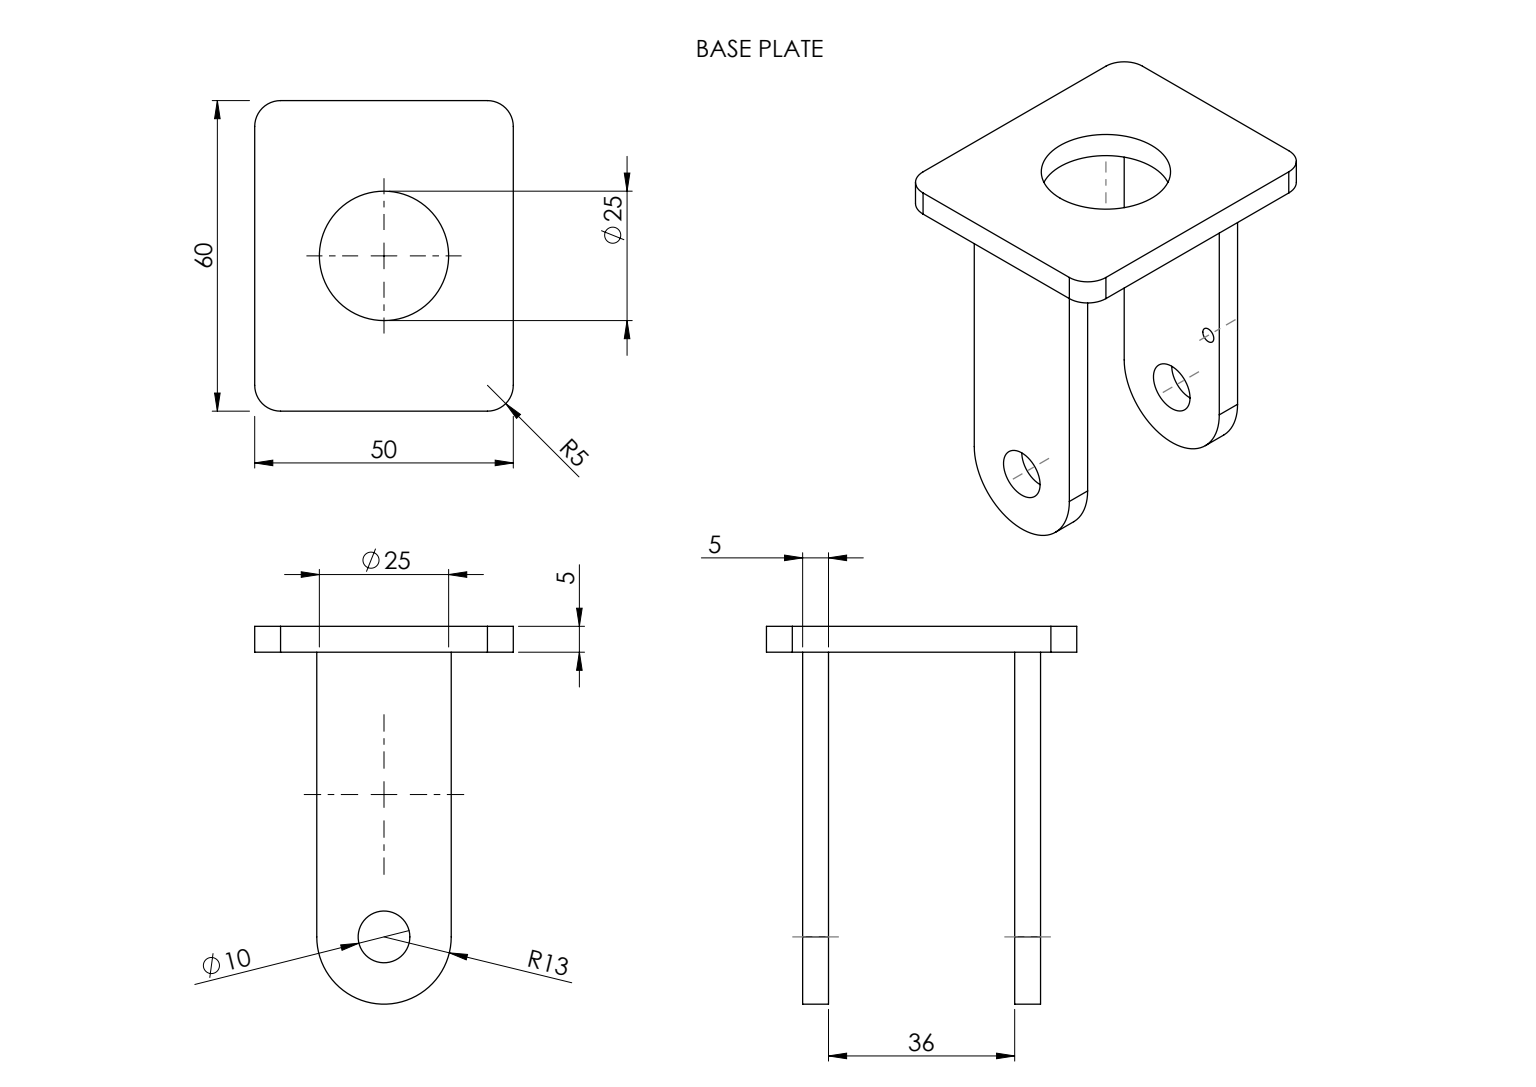
ISO-10303-21;
HEADER;
FILE_DESCRIPTION (('STEP AP214'),
    '1' );
FILE_NAME ('base plate.step',
    '2026-09-30T16:28:02',
    ( '' ),
    ( '' ),
    'SwSTEP 2.0',
    'SolidWorks 2026',
    '' );
FILE_SCHEMA (( 'AUTOMOTIVE_DESIGN' ));
ENDSEC;

DATA;
#4=PLANE ( 'NONE',  #18463 ) ;
#89=DIRECTION ( 'NONE',  ( -1.000000000000000000, 2.207829878515935943E-16, 0.000000000000000000 ) ) ;
#94=CARTESIAN_POINT ( 'NONE',  ( -13.00000000000001243, 55.00000000000000711, 18.00000000000000000 ) ) ;
#112=AXIS2_PLACEMENT_3D ( 'NONE', #25183, #25333, #20434 ) ;
#150=DIRECTION ( 'NONE',  ( 0.000000000000000000, -0.000000000000000000, -1.000000000000000000 ) ) ;
#243=( NAMED_UNIT ( * ) PLANE_ANGLE_UNIT ( ) SI_UNIT ( $, .RADIAN. ) );
#303=EDGE_CURVE ( 'NONE', #13765, #18617, #4330, .T. ) ;
#312=ORIENTED_EDGE ( 'NONE', *, *, #15522, .T. ) ;
#351=PLANE ( 'NONE',  #28566 ) ;
#361=DIRECTION ( 'NONE',  ( 0.000000000000000000, -1.000000000000000000, 0.000000000000000000 ) ) ;
#433=CARTESIAN_POINT ( 'NONE',  ( -13.00000000000001243, 55.00000000000000711, -23.00000000000000000 ) ) ;
#466=ORIENTED_EDGE ( 'NONE', *, *, #9296, .T. ) ;
#467=EDGE_CURVE ( 'NONE', #22249, #23534, #732, .T. ) ;
#553=DIRECTION ( 'NONE',  ( -0.000000000000000000, -1.000000000000000000, -0.000000000000000000 ) ) ;
#578=AXIS2_PLACEMENT_3D ( 'NONE', #20455, #15424, #27383 ) ;
#597=DIRECTION ( 'NONE',  ( -2.207829878515935943E-16, 1.000000000000000000, 0.000000000000000000 ) ) ;
#643=DIRECTION ( 'NONE',  ( 0.000000000000000000, -1.000000000000000000, 0.000000000000000000 ) ) ;
#651=ORIENTED_EDGE ( 'NONE', *, *, #17517, .T. ) ;
#653=VERTEX_POINT ( 'NONE', #12872 ) ;
#675=DIRECTION ( 'NONE',  ( -0.000000000000000000, 1.000000000000000000, -0.000000000000000000 ) ) ;
#732=LINE ( 'NONE', #12472, #2865 ) ;
#752=CARTESIAN_POINT ( 'NONE',  ( 19.99999999999998934, 55.00000000000000711, -30.00000000000000000 ) ) ;
#753=ORIENTED_EDGE ( 'NONE', *, *, #7733, .T. ) ;
#775=EDGE_CURVE ( 'NONE', #20254, #13743, #1148, .T. ) ;
#790=CARTESIAN_POINT ( 'NONE',  ( 0.000000000000000000, 0.000000000000000000, 23.00000000000000000 ) ) ;
#820=AXIS2_PLACEMENT_3D ( 'NONE', #9199, #2219, #20356 ) ;
#827=AXIS2_PLACEMENT_3D ( 'NONE', #15460, #13176, #18050 ) ;
#846=VERTEX_POINT ( 'NONE', #9130 ) ;
#852=ORIENTED_EDGE ( 'NONE', *, *, #16824, .T. ) ;
#873=DIRECTION ( 'NONE',  ( 0.000000000000000000, 0.000000000000000000, 1.000000000000000000 ) ) ;
#883=CARTESIAN_POINT ( 'NONE',  ( -24.99999999999999289, 60.00000000000000711, -30.00000000000000711 ) ) ;
#951=EDGE_CURVE ( 'NONE', #20254, #12966, #17007, .T. ) ;
#1021=( NAMED_UNIT ( * ) PLANE_ANGLE_UNIT ( ) SI_UNIT ( $, .RADIAN. ) );
#1050=ORIENTED_EDGE ( 'NONE', *, *, #15240, .T. ) ;
#1103=VECTOR ( 'NONE', #29704, 1000.000000000000000 ) ;
#1148=LINE ( 'NONE', #3294, #1929 ) ;
#1209=DIRECTION ( 'NONE',  ( -1.387778780781445922E-16, 0.000000000000000000, 1.000000000000000000 ) ) ;
#1239=EDGE_CURVE ( 'NONE', #12966, #20254, #11655, .T. ) ;
#1281=DIRECTION ( 'NONE',  ( -0.000000000000000000, -0.000000000000000000, 1.000000000000000000 ) ) ;
#1304=ADVANCED_FACE ( 'NONE', ( #10036 ), #15218, .F. ) ;
#1305=ORIENTED_EDGE ( 'NONE', *, *, #467, .F. ) ;
#1362=FACE_OUTER_BOUND ( 'NONE', #5538, .T. ) ;
#1413=CARTESIAN_POINT ( 'NONE',  ( 20.00000000000000711, 60.00000000000000711, 29.99999999999998579 ) ) ;
#1433=CARTESIAN_POINT ( 'NONE',  ( 0.000000000000000000, 0.000000000000000000, -23.00000000000000000 ) ) ;
#1502=EDGE_LOOP ( 'NONE', ( #15115, #4598, #15245, #10391 ) ) ;
#1512=AXIS2_PLACEMENT_3D ( 'NONE', #12480, #12790, #7761 ) ;
#1514=LINE ( 'NONE', #20110, #6493 ) ;
#1535=PLANE ( 'NONE',  #25718 ) ;
#1601=LINE ( 'NONE', #10877, #8584 ) ;
#1665=EDGE_CURVE ( 'NONE', #3391, #13743, #22398, .T. ) ;
#1666=CARTESIAN_POINT ( 'NONE',  ( -24.99999999999998934, 55.00000000000000711, 29.99999999999999289 ) ) ;
#1684=LINE ( 'NONE', #13564, #22276 ) ;
#1775=VECTOR ( 'NONE', #13954, 1000.000000000000000 ) ;
#1791=DIRECTION ( 'NONE',  ( -0.000000000000000000, 1.000000000000000000, -0.000000000000000000 ) ) ;
#1812=CARTESIAN_POINT ( 'NONE',  ( -24.99999999999998934, 55.00000000000000711, 24.99999999999998934 ) ) ;
#1837=EDGE_CURVE ( 'NONE', #23534, #6999, #8618, .T. ) ;
#1921=CARTESIAN_POINT ( 'NONE',  ( -19.99999999999998934, 60.00000000000000711, 29.99999999999999289 ) ) ;
#1928=LINE ( 'NONE', #13648, #29476 ) ;
#1929=VECTOR ( 'NONE', #5267, 1000.000000000000000 ) ;
#1988=CARTESIAN_POINT ( 'NONE',  ( 8.469702402841419307E-15, 55.00000000000000711, 12.49999999999999112 ) ) ;
#2054=DIRECTION ( 'NONE',  ( 0.000000000000000000, 0.000000000000000000, -1.000000000000000000 ) ) ;
#2059=ORIENTED_EDGE ( 'NONE', *, *, #8323, .T. ) ;
#2102=AXIS2_PLACEMENT_3D ( 'NONE', #21046, #150, #16913 ) ;
#2147=DIRECTION ( 'NONE',  ( 0.000000000000000000, 0.000000000000000000, -1.000000000000000000 ) ) ;
#2163=ORIENTED_EDGE ( 'NONE', *, *, #14056, .F. ) ;
#2218=EDGE_CURVE ( 'NONE', #19798, #4416, #26479, .T. ) ;
#2219=DIRECTION ( 'NONE',  ( 0.000000000000000000, -1.000000000000000000, 0.000000000000000000 ) ) ;
#2237=( LENGTH_UNIT ( ) NAMED_UNIT ( * ) SI_UNIT ( .MILLI., .METRE. ) );
#2268=AXIS2_PLACEMENT_3D ( 'NONE', #28367, #7860, #2691 ) ;
#2305=ADVANCED_FACE ( 'NONE', ( #10419 ), #19581, .F. ) ;
#2341=DIRECTION ( 'NONE',  ( -1.000000000000000000, 0.000000000000000000, 1.387778780781445676E-16 ) ) ;
#2364=CYLINDRICAL_SURFACE ( 'NONE', #20773, 13.00000000000000178 ) ;
#2387=ADVANCED_FACE ( 'NONE', ( #8725 ), #10727, .F. ) ;
#2401=CARTESIAN_POINT ( 'NONE',  ( 13.00000000000001243, 55.00000000000000711, 18.00000000000000000 ) ) ;
#2495=EDGE_CURVE ( 'NONE', #18617, #28674, #20327, .T. ) ;
#2518=CARTESIAN_POINT ( 'NONE',  ( -13.00000000000000178, -2.870178842070716726E-15, -18.00000000000000000 ) ) ;
#2527=CARTESIAN_POINT ( 'NONE',  ( 0.000000000000000000, 0.000000000000000000, -23.00000000000000000 ) ) ;
#2554=ORIENTED_EDGE ( 'NONE', *, *, #28546, .F. ) ;
#2586=CIRCLE ( 'NONE', #11332, 5.000000000000000888 ) ;
#2630=DIRECTION ( 'NONE',  ( -1.000000000000000000, -2.207829878515935943E-16, 0.000000000000000000 ) ) ;
#2640=FACE_BOUND ( 'NONE', #22846, .T. ) ;
#2691=DIRECTION ( 'NONE',  ( 6.938893903907226800E-15, 0.000000000000000000, -1.000000000000000000 ) ) ;
#2739=VECTOR ( 'NONE', #10171, 1000.000000000000000 ) ;
#2788=CIRCLE ( 'NONE', #23227, 5.000000000000000000 ) ;
#2793=DIRECTION ( 'NONE',  ( -0.000000000000000000, 0.000000000000000000, 1.000000000000000000 ) ) ;
#2865=VECTOR ( 'NONE', #597, 1000.000000000000000 ) ;
#2897=ADVANCED_FACE ( 'NONE', ( #26440 ), #17257, .T. ) ;
#2982=DIRECTION ( 'NONE',  ( 0.000000000000000000, 0.000000000000000000, -1.000000000000000000 ) ) ;
#2988=CARTESIAN_POINT ( 'NONE',  ( 13.00000000000000178, -2.870178842070716726E-15, 23.00000000000000000 ) ) ;
#3027=DIRECTION ( 'NONE',  ( 0.000000000000000000, -1.000000000000000000, -0.000000000000000000 ) ) ;
#3040=ADVANCED_FACE ( 'NONE', ( #7024, #21193 ), #4, .F. ) ;
#3047=DIRECTION ( 'NONE',  ( 1.000000000000000000, 0.000000000000000000, 0.000000000000000000 ) ) ;
#3050=DIRECTION ( 'NONE',  ( 0.000000000000000000, -1.000000000000000000, 0.000000000000000000 ) ) ;
#3065=CARTESIAN_POINT ( 'NONE',  ( 13.00000000000001243, 55.00000000000000711, -23.00000000000000000 ) ) ;
#3163=( LENGTH_UNIT ( ) NAMED_UNIT ( * ) SI_UNIT ( .MILLI., .METRE. ) );
#3232=PRODUCT_CONTEXT ( 'NONE', #11423, 'mechanical' ) ;
#3236=COLOUR_RGB ( '', 0.09019608, 0.27058824, 0.51372549) ;
#3274=AXIS2_PLACEMENT_3D ( 'NONE', #13005, #17580, #15441 ) ;
#3285=CARTESIAN_POINT ( 'NONE',  ( -5.000000000000000000, 0.000000000000000000, -23.00000000000000000 ) ) ;
#3291=ORIENTED_EDGE ( 'NONE', *, *, #21767, .F. ) ;
#3294=CARTESIAN_POINT ( 'NONE',  ( 8.469702402841419307E-15, 60.00000000000000711, 12.49999999999999112 ) ) ;
#3295=LINE ( 'NONE', #19892, #25365 ) ;
#3296=CIRCLE ( 'NONE', #20319, 1.499999999999996225 ) ;
#3349=LINE ( 'NONE', #10189, #11351 ) ;
#3350=CARTESIAN_POINT ( 'NONE',  ( 6.938893903907228378E-15, 60.00000000000000711, -1.040834085586084257E-14 ) ) ;
#3369=ORIENTED_EDGE ( 'NONE', *, *, #4832, .F. ) ;
#3391=VERTEX_POINT ( 'NONE', #24824 ) ;
#3430=DIRECTION ( 'NONE',  ( 1.000000000000000000, 0.000000000000000000, 0.000000000000000000 ) ) ;
#3463=DIRECTION ( 'NONE',  ( 1.000000000000000000, 0.000000000000000000, 0.000000000000000000 ) ) ;
#3477=ADVANCED_FACE ( 'NONE', ( #25560 ), #5110, .F. ) ;
#3497=DIRECTION ( 'NONE',  ( 1.000000000000000000, 0.000000000000000000, 1.387778780781445922E-16 ) ) ;
#3515=CARTESIAN_POINT ( 'NONE',  ( 13.00000000000000178, -2.870178842070716726E-15, 23.00000000000000000 ) ) ;
#3527=VECTOR ( 'NONE', #675, 1000.000000000000000 ) ;
#3535=ORIENTED_EDGE ( 'NONE', *, *, #29533, .T. ) ;
#3543=AXIS2_PLACEMENT_3D ( 'NONE', #15895, #13310, #22633 ) ;
#3550=EDGE_LOOP ( 'NONE', ( #25606, #8516, #3369, #29957 ) ) ;
#3565=ORIENTED_EDGE ( 'NONE', *, *, #25043, .T. ) ;
#3584=LINE ( 'NONE', #22188, #8766 ) ;
#3613=CARTESIAN_POINT ( 'NONE',  ( 10.00000000000008527, 17.32050807568872486, -30.00000000000000711 ) ) ;
#3645=EDGE_CURVE ( 'NONE', #27580, #29940, #3295, .T. ) ;
#3670=CARTESIAN_POINT ( 'NONE',  ( -13.00000000000001243, 55.00000000000000711, 23.00000000000000000 ) ) ;
#3687=ORIENTED_EDGE ( 'NONE', *, *, #24489, .F. ) ;
#3776=CARTESIAN_POINT ( 'NONE',  ( -13.00000000000000178, -2.870178842070716726E-15, -18.00000000000000000 ) ) ;
#3785=ADVANCED_FACE ( 'NONE', ( #11184 ), #8445, .T. ) ;
#3815=DIRECTION ( 'NONE',  ( -0.000000000000000000, 1.000000000000000000, -0.000000000000000000 ) ) ;
#3841=CARTESIAN_POINT ( 'NONE',  ( 25.00000000000000000, 55.00000000000000711, -24.99999999999999289 ) ) ;
#3862=EDGE_CURVE ( 'NONE', #15686, #5157, #11281, .T. ) ;
#3942=( GEOMETRIC_REPRESENTATION_CONTEXT ( 3 ) GLOBAL_UNCERTAINTY_ASSIGNED_CONTEXT ( ( #30012 ) ) GLOBAL_UNIT_ASSIGNED_CONTEXT ( ( #3163, #10603, #21756 ) ) REPRESENTATION_CONTEXT ( 'NONE', 'WORKASPACE' ) );
#3978=DIRECTION ( 'NONE',  ( -0.000000000000000000, -0.000000000000000000, 1.000000000000000000 ) ) ;
#3985=VERTEX_POINT ( 'NONE', #10993 ) ;
#3989=EDGE_CURVE ( 'NONE', #13765, #14128, #27497, .T. ) ;
#4003=VECTOR ( 'NONE', #1281, 1000.000000000000000 ) ;
#4052=EDGE_LOOP ( 'NONE', ( #28141, #29867, #12630, #29986 ) ) ;
#4093=DIRECTION ( 'NONE',  ( 1.000000000000000000, 0.000000000000000000, -1.387778780781445676E-16 ) ) ;
#4112=DIRECTION ( 'NONE',  ( -0.000000000000000000, -0.000000000000000000, 1.000000000000000000 ) ) ;
#4160=EDGE_CURVE ( 'NONE', #13649, #22275, #16289, .T. ) ;
#4162=ORIENTED_EDGE ( 'NONE', *, *, #15722, .T. ) ;
#4184=ADVANCED_FACE ( 'NONE', ( #11711 ), #18889, .F. ) ;
#4330=CIRCLE ( 'NONE', #21386, 13.00000000000000178 ) ;
#4372=VECTOR ( 'NONE', #5031, 1000.000000000000000 ) ;
#4393=VECTOR ( 'NONE', #13496, 1000.000000000000000 ) ;
#4416=VERTEX_POINT ( 'NONE', #26691 ) ;
#4431=CARTESIAN_POINT ( 'NONE',  ( 0.000000000000000000, 0.000000000000000000, 18.00000000000000000 ) ) ;
#4432=CARTESIAN_POINT ( 'NONE',  ( 13.00000000000001243, 55.00000000000000711, -23.00000000000000000 ) ) ;
#4500=CARTESIAN_POINT ( 'NONE',  ( -24.99999999999998934, 55.00000000000000711, 29.99999999999999289 ) ) ;
#4511=SURFACE_STYLE_FILL_AREA ( #18392 ) ;
#4521=FACE_BOUND ( 'NONE', #26367, .T. ) ;
#4598=ORIENTED_EDGE ( 'NONE', *, *, #12300, .F. ) ;
#4649=CIRCLE ( 'NONE', #19739, 1.499999999999996225 ) ;
#4662=ADVANCED_FACE ( 'NONE', ( #7137, #23312 ), #23468, .F. ) ;
#4688=DIRECTION ( 'NONE',  ( 0.000000000000000000, 0.000000000000000000, -1.000000000000000000 ) ) ;
#4708=AXIS2_PLACEMENT_3D ( 'NONE', #17140, #9953, #14831 ) ;
#4743=CARTESIAN_POINT ( 'NONE',  ( -24.99999999999999289, 60.00000000000000711, -25.00000000000000000 ) ) ;
#4832=EDGE_CURVE ( 'NONE', #17767, #27247, #22973, .T. ) ;
#4914=CARTESIAN_POINT ( 'NONE',  ( -13.00000000000000178, -2.870178842070716726E-15, 23.00000000000000000 ) ) ;
#4918=AXIS2_PLACEMENT_3D ( 'NONE', #23936, #3027, #22224 ) ;
#5008=VERTEX_POINT ( 'NONE', #15798 ) ;
#5031=DIRECTION ( 'NONE',  ( -0.000000000000000000, -0.000000000000000000, 1.000000000000000000 ) ) ;
#5066=LINE ( 'NONE', #7371, #17270 ) ;
#5110=PLANE ( 'NONE',  #21390 ) ;
#5157=VERTEX_POINT ( 'NONE', #22542 ) ;
#5205=CARTESIAN_POINT ( 'NONE',  ( 13.00000000000001243, 55.00000000000000711, 23.00000000000000000 ) ) ;
#5217=DIRECTION ( 'NONE',  ( -2.207829878515935943E-16, 1.000000000000000000, 0.000000000000000000 ) ) ;
#5267=DIRECTION ( 'NONE',  ( -0.000000000000000000, -1.000000000000000000, -0.000000000000000000 ) ) ;
#5435=CARTESIAN_POINT ( 'NONE',  ( 0.000000000000000000, 0.000000000000000000, 0.000000000000000000 ) ) ;
#5478=CIRCLE ( 'NONE', #16208, 12.50000000000000000 ) ;
#5480=DIRECTION ( 'NONE',  ( 1.000000000000000000, 0.000000000000000000, 0.000000000000000000 ) ) ;
#5538=EDGE_LOOP ( 'NONE', ( #1050, #25690, #2554, #15574 ) ) ;
#5549=ADVANCED_FACE ( 'NONE', ( #17306 ), #19296, .F. ) ;
#5552=CYLINDRICAL_SURFACE ( 'NONE', #4708, 12.50000000000000000 ) ;
#5570=CARTESIAN_POINT ( 'NONE',  ( 25.00000000000001066, 60.00000000000000711, 24.99999999999998579 ) ) ;
#5587=SURFACE_STYLE_FILL_AREA ( #26505 ) ;
#5591=ORIENTED_EDGE ( 'NONE', *, *, #11689, .F. ) ;
#5615=EDGE_LOOP ( 'NONE', ( #18841, #13481, #20447, #14888 ) ) ;
#5647=ORIENTED_EDGE ( 'NONE', *, *, #26563, .F. ) ;
#5650=CARTESIAN_POINT ( 'NONE',  ( 13.00000000000000178, -2.870178842070716726E-15, -23.00000000000000000 ) ) ;
#5705=DIRECTION ( 'NONE',  ( 0.000000000000000000, 0.000000000000000000, -1.000000000000000000 ) ) ;
#5706=VECTOR ( 'NONE', #21523, 1000.000000000000000 ) ;
#5713=EDGE_CURVE ( 'NONE', #15063, #11701, #3584, .T. ) ;
#5752=ADVANCED_FACE ( 'NONE', ( #14067 ), #25532, .T. ) ;
#5783=CARTESIAN_POINT ( 'NONE',  ( 0.000000000000000000, 0.000000000000000000, 18.00000000000000000 ) ) ;
#5798=CARTESIAN_POINT ( 'NONE',  ( 0.000000000000000000, 0.000000000000000000, -23.00000000000000000 ) ) ;
#5808=ORIENTED_EDGE ( 'NONE', *, *, #14056, .T. ) ;
#5824=DIRECTION ( 'NONE',  ( -0.000000000000000000, -0.000000000000000000, -1.000000000000000000 ) ) ;
#5883=( GEOMETRIC_REPRESENTATION_CONTEXT ( 3 ) GLOBAL_UNCERTAINTY_ASSIGNED_CONTEXT ( ( #25378 ) ) GLOBAL_UNIT_ASSIGNED_CONTEXT ( ( #17320, #1021, #22364 ) ) REPRESENTATION_CONTEXT ( 'NONE', 'WORKASPACE' ) );
#5908=CARTESIAN_POINT ( 'NONE',  ( 13.00000000000000178, -2.870178842070716726E-15, 18.00000000000000000 ) ) ;
#5989=EDGE_LOOP ( 'NONE', ( #19822, #11466, #753, #3565 ) ) ;
#6015=DIRECTION ( 'NONE',  ( -0.000000000000000000, -0.000000000000000000, -1.000000000000000000 ) ) ;
#6114=ORIENTED_EDGE ( 'NONE', *, *, #18133, .T. ) ;
#6118=EDGE_LOOP ( 'NONE', ( #27463, #20840, #21549, #13025 ) ) ;
#6126=EDGE_LOOP ( 'NONE', ( #14213, #22314, #11910, #19662 ) ) ;
#6159=VECTOR ( 'NONE', #28472, 1000.000000000000000 ) ;
#6170=DIRECTION ( 'NONE',  ( 1.000000000000000000, 0.000000000000000000, -1.387778780781445676E-16 ) ) ;
#6378=AXIS2_PLACEMENT_3D ( 'NONE', #23617, #16138, #4688 ) ;
#6493=VECTOR ( 'NONE', #29490, 1000.000000000000000 ) ;
#6515=ORIENTED_EDGE ( 'NONE', *, *, #10062, .T. ) ;
#6572=EDGE_LOOP ( 'NONE', ( #8098, #6114, #7686, #28054 ) ) ;
#6704=CARTESIAN_POINT ( 'NONE',  ( -13.00000000000000178, -2.870178842070716726E-15, -23.00000000000000000 ) ) ;
#6725=AXIS2_PLACEMENT_3D ( 'NONE', #19230, #2630, #23369 ) ;
#6739=DIRECTION ( 'NONE',  ( -0.000000000000000000, 1.000000000000000000, 0.000000000000000000 ) ) ;
#6762=LINE ( 'NONE', #18196, #20456 ) ;
#6765=FACE_OUTER_BOUND ( 'NONE', #29980, .T. ) ;
#6810=LINE ( 'NONE', #8780, #29821 ) ;
#6824=AXIS2_PLACEMENT_3D ( 'NONE', #3350, #24399, #7910 ) ;
#6906=CARTESIAN_POINT ( 'NONE',  ( -13.00000000000000178, -2.870178842070716726E-15, -23.00000000000000000 ) ) ;
#6959=SURFACE_STYLE_USAGE ( .BOTH. , #9066 ) ;
#6999=VERTEX_POINT ( 'NONE', #2401 ) ;
#7024=FACE_OUTER_BOUND ( 'NONE', #25518, .T. ) ;
#7050=AXIS2_PLACEMENT_3D ( 'NONE', #11624, #14060, #13909 ) ;
#7108=ORIENTED_EDGE ( 'NONE', *, *, #3989, .T. ) ;
#7137=FACE_OUTER_BOUND ( 'NONE', #13454, .T. ) ;
#7222=VERTEX_POINT ( 'NONE', #7714 ) ;
#7235=ADVANCED_FACE ( 'NONE', ( #17023 ), #28514, .F. ) ;
#7241=CARTESIAN_POINT ( 'NONE',  ( 0.000000000000000000, 0.000000000000000000, 23.00000000000000000 ) ) ;
#7259=DIRECTION ( 'NONE',  ( -2.207829878515935943E-16, -1.000000000000000000, 0.000000000000000000 ) ) ;
#7269=VERTEX_POINT ( 'NONE', #10892 ) ;
#7365=FACE_OUTER_BOUND ( 'NONE', #30006, .T. ) ;
#7371=CARTESIAN_POINT ( 'NONE',  ( 0.000000000000000000, 55.00000000000000711, -18.00000000000000000 ) ) ;
#7417=LINE ( 'NONE', #14557, #9015 ) ;
#7451=VECTOR ( 'NONE', #14383, 1000.000000000000000 ) ;
#7520=DIRECTION ( 'NONE',  ( -1.000000000000000000, 0.000000000000000000, 0.000000000000000000 ) ) ;
#7563=CARTESIAN_POINT ( 'NONE',  ( -24.99999999999998934, 60.00000000000000711, 29.99999999999999289 ) ) ;
#7578=DIRECTION ( 'NONE',  ( 0.000000000000000000, 0.000000000000000000, 1.000000000000000000 ) ) ;
#7673=ORIENTED_EDGE ( 'NONE', *, *, #26824, .F. ) ;
#7686=ORIENTED_EDGE ( 'NONE', *, *, #22977, .T. ) ;
#7714=CARTESIAN_POINT ( 'NONE',  ( 5.000000000000000000, -6.123233995736766282E-16, -23.00000000000000000 ) ) ;
#7717=ORIENTED_EDGE ( 'NONE', *, *, #10620, .F. ) ;
#7733=EDGE_CURVE ( 'NONE', #13894, #27247, #16389, .T. ) ;
#7761=DIRECTION ( 'NONE',  ( -1.000000000000000000, 0.000000000000000000, 0.000000000000000000 ) ) ;
#7773=LINE ( 'NONE', #3065, #4372 ) ;
#7832=FACE_OUTER_BOUND ( 'NONE', #23497, .T. ) ;
#7860=DIRECTION ( 'NONE',  ( -0.000000000000000000, 1.000000000000000000, 0.000000000000000000 ) ) ;
#7894=AXIS2_PLACEMENT_3D ( 'NONE', #1433, #5705, #19876 ) ;
#7910=DIRECTION ( 'NONE',  ( 0.000000000000000000, 0.000000000000000000, 1.000000000000000000 ) ) ;
#7942=VECTOR ( 'NONE', #4093, 1000.000000000000000 ) ;
#7943=EDGE_CURVE ( 'NONE', #846, #11701, #16545, .T. ) ;
#8000=VERTEX_POINT ( 'NONE', #28946 ) ;
#8015=EDGE_CURVE ( 'NONE', #27929, #29924, #24778, .T. ) ;
#8034=EDGE_CURVE ( 'NONE', #7222, #27929, #20072, .T. ) ;
#8053=CARTESIAN_POINT ( 'NONE',  ( -19.99999999999999645, 55.00000000000000711, -30.00000000000000711 ) ) ;
#8054=CARTESIAN_POINT ( 'NONE',  ( 13.00000000000000178, -2.870178842070716726E-15, -23.00000000000000000 ) ) ;
#8098=ORIENTED_EDGE ( 'NONE', *, *, #10062, .F. ) ;
#8101=CIRCLE ( 'NONE', #25184, 5.000000000000000888 ) ;
#8125=ORIENTED_EDGE ( 'NONE', *, *, #2218, .T. ) ;
#8171=DIRECTION ( 'NONE',  ( 0.000000000000000000, 0.000000000000000000, -1.000000000000000000 ) ) ;
#8238=ADVANCED_FACE ( 'NONE', ( #13455 ), #30007, .F. ) ;
#8280=EDGE_CURVE ( 'NONE', #13743, #3391, #5478, .T. ) ;
#8313=FILL_AREA_STYLE_COLOUR ( '', #13662 ) ;
#8323=EDGE_CURVE ( 'NONE', #11701, #27580, #23047, .T. ) ;
#8376=DIRECTION ( 'NONE',  ( -1.000000000000000000, 0.000000000000000000, 1.734723475976807587E-16 ) ) ;
#8424=FACE_OUTER_BOUND ( 'NONE', #21010, .T. ) ;
#8445=CYLINDRICAL_SURFACE ( 'NONE', #9821, 13.00000000000000178 ) ;
#8516=ORIENTED_EDGE ( 'NONE', *, *, #25043, .F. ) ;
#8575=DIRECTION ( 'NONE',  ( 0.000000000000000000, 0.000000000000000000, 1.000000000000000000 ) ) ;
#8579=CARTESIAN_POINT ( 'NONE',  ( 13.00000000000000178, -2.870178842070716726E-15, -23.00000000000000000 ) ) ;
#8584=VECTOR ( 'NONE', #6015, 1000.000000000000000 ) ;
#8615=AXIS2_PLACEMENT_3D ( 'NONE', #19727, #29096, #17150 ) ;
#8618=LINE ( 'NONE', #27583, #28799 ) ;
#8696=DIRECTION ( 'NONE',  ( 0.000000000000000000, 0.000000000000000000, -1.000000000000000000 ) ) ;
#8718=CLOSED_SHELL ( 'NONE', ( #9615, #30063, #5549, #2387, #15377, #3785, #3477, #23204, #20365, #3040, #22166, #4662, #12438, #1304, #7235, #8238, #15208, #26364, #24022, #2305, #12214, #14305, #27399, #5752, #15087, #21129, #2897, #4184 ) ) ;
#8725=FACE_OUTER_BOUND ( 'NONE', #5615, .T. ) ;
#8766=VECTOR ( 'NONE', #6170, 1000.000000000000000 ) ;
#8780=CARTESIAN_POINT ( 'NONE',  ( 25.00000000000000000, 60.00000000000000711, -24.99999999999999289 ) ) ;
#8807=ORIENTED_EDGE ( 'NONE', *, *, #17517, .F. ) ;
#8869=EDGE_CURVE ( 'NONE', #14718, #29543, #24509, .T. ) ;
#8877=DIRECTION ( 'NONE',  ( 0.000000000000000000, 1.000000000000000000, 0.000000000000000000 ) ) ;
#8951=EDGE_CURVE ( 'NONE', #29592, #22249, #3349, .T. ) ;
#8975=DIRECTION ( 'NONE',  ( 0.000000000000000000, -1.000000000000000000, -0.000000000000000000 ) ) ;
#9015=VECTOR ( 'NONE', #23904, 1000.000000000000000 ) ;
#9030=MECHANICAL_DESIGN_GEOMETRIC_PRESENTATION_REPRESENTATION('',(#17819),#16345);
#9049=CIRCLE ( 'NONE', #2268, 5.000000000000000888 ) ;
#9066=SURFACE_SIDE_STYLE ('',( #4511 ) ) ;
#9100=DIRECTION ( 'NONE',  ( 1.000000000000000000, 0.000000000000000000, 0.000000000000000000 ) ) ;
#9130=CARTESIAN_POINT ( 'NONE',  ( 20.00000000000000711, 55.00000000000000711, 29.99999999999998579 ) ) ;
#9164=AXIS2_PLACEMENT_3D ( 'NONE', #29513, #8975, #13115 ) ;
#9171=DIRECTION ( 'NONE',  ( 0.000000000000000000, 0.000000000000000000, 1.000000000000000000 ) ) ;
#9199=CARTESIAN_POINT ( 'NONE',  ( 20.00000000000000355, 60.00000000000000711, -24.99999999999999645 ) ) ;
#9209=AXIS2_PLACEMENT_3D ( 'NONE', #12150, #9859, #7578 ) ;
#9221=EDGE_LOOP ( 'NONE', ( #25685, #14817, #2163, #24551 ) ) ;
#9249=CARTESIAN_POINT ( 'NONE',  ( 0.000000000000000000, 0.000000000000000000, -18.00000000000000000 ) ) ;
#9296=EDGE_CURVE ( 'NONE', #14128, #18267, #11205, .T. ) ;
#9370=CARTESIAN_POINT ( 'NONE',  ( 13.00000000000000178, -2.870178842070716726E-15, 23.00000000000000000 ) ) ;
#9466=VECTOR ( 'NONE', #5824, 1000.000000000000000 ) ;
#9483=ORIENTED_EDGE ( 'NONE', *, *, #21561, .T. ) ;
#9499=ORIENTED_EDGE ( 'NONE', *, *, #10958, .T. ) ;
#9566=DIRECTION ( 'NONE',  ( -0.000000000000000000, -0.000000000000000000, 1.000000000000000000 ) ) ;
#9615=ADVANCED_FACE ( 'NONE', ( #24674 ), #22380, .F. ) ;
#9745=ORIENTED_EDGE ( 'NONE', *, *, #8869, .F. ) ;
#9748=ORIENTED_EDGE ( 'NONE', *, *, #20237, .F. ) ;
#9800=EDGE_CURVE ( 'NONE', #12966, #3391, #6762, .T. ) ;
#9817=CARTESIAN_POINT ( 'NONE',  ( -19.99999999999999289, 55.00000000000000711, -25.00000000000000000 ) ) ;
#9821=AXIS2_PLACEMENT_3D ( 'NONE', #15907, #10880, #13468 ) ;
#9853=ORIENTED_EDGE ( 'NONE', *, *, #15130, .T. ) ;
#9859=DIRECTION ( 'NONE',  ( 0.000000000000000000, 1.000000000000000000, 0.000000000000000000 ) ) ;
#9873=CARTESIAN_POINT ( 'NONE',  ( -24.99999999999999289, 55.00000000000000711, -25.00000000000000000 ) ) ;
#9908=DIRECTION ( 'NONE',  ( -0.000000000000000000, -0.000000000000000000, 1.000000000000000000 ) ) ;
#9917=PLANE ( 'NONE',  #6725 ) ;
#9942=CARTESIAN_POINT ( 'NONE',  ( 10.00000000000008527, 17.32050807568872486, -17.99999999999999645 ) ) ;
#9953=DIRECTION ( 'NONE',  ( -0.000000000000000000, -1.000000000000000000, -0.000000000000000000 ) ) ;
#9968=EDGE_CURVE ( 'NONE', #22275, #25189, #5066, .T. ) ;
#9987=DIRECTION ( 'NONE',  ( -5.782411586589357392E-17, 0.000000000000000000, -1.000000000000000000 ) ) ;
#10036=FACE_OUTER_BOUND ( 'NONE', #9221, .T. ) ;
#10062=EDGE_CURVE ( 'NONE', #8000, #7269, #16283, .T. ) ;
#10141=EDGE_CURVE ( 'NONE', #15686, #14718, #28919, .T. ) ;
#10147=SURFACE_SIDE_STYLE ('',( #5587 ) ) ;
#10171=DIRECTION ( 'NONE',  ( -1.000000000000000000, -0.000000000000000000, -1.387778780781445922E-16 ) ) ;
#10176=VERTEX_POINT ( 'NONE', #14960 ) ;
#10189=CARTESIAN_POINT ( 'NONE',  ( -13.00000000000000178, -2.870178842070716726E-15, 23.00000000000000000 ) ) ;
#10192=ORIENTED_EDGE ( 'NONE', *, *, #12719, .T. ) ;
#10204=VERTEX_POINT ( 'NONE', #14806 ) ;
#10304=CARTESIAN_POINT ( 'NONE',  ( 25.00000000000001066, 60.00000000000000711, 24.99999999999998579 ) ) ;
#10386=DIRECTION ( 'NONE',  ( -0.000000000000000000, -0.000000000000000000, 1.000000000000000000 ) ) ;
#10391=ORIENTED_EDGE ( 'NONE', *, *, #28844, .T. ) ;
#10419=FACE_OUTER_BOUND ( 'NONE', #1502, .T. ) ;
#10446=DIRECTION ( 'NONE',  ( 1.000000000000000000, 0.000000000000000000, 0.000000000000000000 ) ) ;
#10507=LINE ( 'NONE', #5650, #11093 ) ;
#10591=ORIENTED_EDGE ( 'NONE', *, *, #7943, .F. ) ;
#10603=( NAMED_UNIT ( * ) PLANE_ANGLE_UNIT ( ) SI_UNIT ( $, .RADIAN. ) );
#10620=EDGE_CURVE ( 'NONE', #20836, #6999, #22543, .T. ) ;
#10644=CARTESIAN_POINT ( 'NONE',  ( 0.000000000000000000, 0.000000000000000000, 18.00000000000000000 ) ) ;
#10719=PRODUCT_DEFINITION_FORMATION_WITH_SPECIFIED_SOURCE ( 'ANY', '', #22019, .NOT_KNOWN. ) ;
#10727=CYLINDRICAL_SURFACE ( 'NONE', #25681, 5.000000000000000000 ) ;
#10870=CARTESIAN_POINT ( 'NONE',  ( 0.000000000000000000, 0.000000000000000000, 23.00000000000000000 ) ) ;
#10877=CARTESIAN_POINT ( 'NONE',  ( -13.00000000000001243, 55.00000000000000711, 23.00000000000000000 ) ) ;
#10880=DIRECTION ( 'NONE',  ( -0.000000000000000000, -0.000000000000000000, -1.000000000000000000 ) ) ;
#10892=CARTESIAN_POINT ( 'NONE',  ( 11.50000000000008171, 17.32050807568872486, -23.00000000000000000 ) ) ;
#10950=DIRECTION ( 'NONE',  ( 0.000000000000000000, 0.000000000000000000, -1.000000000000000000 ) ) ;
#10958=EDGE_CURVE ( 'NONE', #13649, #28674, #7417, .T. ) ;
#10966=ORIENTED_EDGE ( 'NONE', *, *, #10620, .T. ) ;
#10993=CARTESIAN_POINT ( 'NONE',  ( -24.99999999999998934, 60.00000000000000711, 24.99999999999998934 ) ) ;
#11011=CARTESIAN_POINT ( 'NONE',  ( 0.000000000000000000, 0.000000000000000000, -23.00000000000000000 ) ) ;
#11093=VECTOR ( 'NONE', #9908, 1000.000000000000000 ) ;
#11170=ORIENTED_EDGE ( 'NONE', *, *, #8015, .T. ) ;
#11184=FACE_OUTER_BOUND ( 'NONE', #26930, .T. ) ;
#11205=CIRCLE ( 'NONE', #18500, 13.00000000000000178 ) ;
#11231=DIRECTION ( 'NONE',  ( -1.000000000000000000, 0.000000000000000000, 0.000000000000000000 ) ) ;
#11281=CIRCLE ( 'NONE', #578, 5.000000000000000000 ) ;
#11332=AXIS2_PLACEMENT_3D ( 'NONE', #9817, #25440, #2982 ) ;
#11351=VECTOR ( 'NONE', #21640, 1000.000000000000000 ) ;
#11406=ORIENTED_EDGE ( 'NONE', *, *, #9800, .T. ) ;
#11423=APPLICATION_CONTEXT ( 'automotive_design' ) ;
#11466=ORIENTED_EDGE ( 'NONE', *, *, #17853, .T. ) ;
#11554=ORIENTED_EDGE ( 'NONE', *, *, #14606, .T. ) ;
#11624=CARTESIAN_POINT ( 'NONE',  ( 10.00000000000008527, 17.32050807568872486, -23.00000000000000000 ) ) ;
#11654=DIRECTION ( 'NONE',  ( 0.000000000000000000, 0.000000000000000000, 1.000000000000000000 ) ) ;
#11655=CIRCLE ( 'NONE', #6824, 12.50000000000000000 ) ;
#11689=EDGE_CURVE ( 'NONE', #653, #5008, #3296, .T. ) ;
#11701=VERTEX_POINT ( 'NONE', #1413 ) ;
#11707=VECTOR ( 'NONE', #9566, 1000.000000000000000 ) ;
#11711=FACE_OUTER_BOUND ( 'NONE', #4052, .T. ) ;
#11744=ORIENTED_EDGE ( 'NONE', *, *, #29533, .F. ) ;
#11761=DIRECTION ( 'NONE',  ( -0.000000000000000000, -0.000000000000000000, -1.000000000000000000 ) ) ;
#11910=ORIENTED_EDGE ( 'NONE', *, *, #10141, .T. ) ;
#12013=CARTESIAN_POINT ( 'NONE',  ( 13.00000000000001243, 55.00000000000000711, -18.00000000000000000 ) ) ;
#12028=VECTOR ( 'NONE', #29870, 1000.000000000000000 ) ;
#12150=CARTESIAN_POINT ( 'NONE',  ( 6.938893903907228378E-15, 55.00000000000000711, -1.040834085586084257E-14 ) ) ;
#12151=EDGE_LOOP ( 'NONE', ( #25845, #6515 ) ) ;
#12155=CIRCLE ( 'NONE', #14110, 5.000000000000000000 ) ;
#12162=CARTESIAN_POINT ( 'NONE',  ( 10.00000000000008527, 17.32050807568872486, -17.99999999999999645 ) ) ;
#12196=EDGE_LOOP ( 'NONE', ( #24533, #466, #24539, #16450 ) ) ;
#12214=ADVANCED_FACE ( 'NONE', ( #21660 ), #17090, .F. ) ;
#12226=CARTESIAN_POINT ( 'NONE',  ( 6.938893903907228378E-15, 60.00000000000000711, -12.50000000000001066 ) ) ;
#12275=DIRECTION ( 'NONE',  ( -1.734723475976807587E-16, 0.000000000000000000, -1.000000000000000000 ) ) ;
#12300=EDGE_CURVE ( 'NONE', #18617, #18267, #10507, .T. ) ;
#12358=DIRECTION ( 'NONE',  ( -1.734723475976807587E-16, 0.000000000000000000, -1.000000000000000000 ) ) ;
#12402=LINE ( 'NONE', #23883, #7451 ) ;
#12420=CARTESIAN_POINT ( 'NONE',  ( 0.000000000000000000, 0.000000000000000000, -18.00000000000000000 ) ) ;
#12438=ADVANCED_FACE ( 'NONE', ( #22432 ), #1535, .F. ) ;
#12472=CARTESIAN_POINT ( 'NONE',  ( -13.00000000000000178, -2.870178842070716726E-15, 18.00000000000000000 ) ) ;
#12480=CARTESIAN_POINT ( 'NONE',  ( 0.000000000000000000, 0.000000000000000000, -23.00000000000000000 ) ) ;
#12487=PRODUCT_DEFINITION_SHAPE ( 'NONE', 'NONE',  #26898 ) ;
#12630=ORIENTED_EDGE ( 'NONE', *, *, #17914, .T. ) ;
#12666=CARTESIAN_POINT ( 'NONE',  ( 13.00000000000000178, -2.870178842070716726E-15, -18.00000000000000000 ) ) ;
#12706=EDGE_LOOP ( 'NONE', ( #13112, #12851, #29450, #7108 ) ) ;
#12719=EDGE_CURVE ( 'NONE', #3985, #15063, #21835, .T. ) ;
#12773=EDGE_LOOP ( 'NONE', ( #13886, #21960, #13814, #21055 ) ) ;
#12790=DIRECTION ( 'NONE',  ( -0.000000000000000000, -0.000000000000000000, 1.000000000000000000 ) ) ;
#12809=LINE ( 'NONE', #3515, #5706 ) ;
#12816=ORIENTED_EDGE ( 'NONE', *, *, #18728, .F. ) ;
#12820=VECTOR ( 'NONE', #16737, 1000.000000000000000 ) ;
#12832=EDGE_LOOP ( 'NONE', ( #16668, #312, #20582, #17458 ) ) ;
#12851=ORIENTED_EDGE ( 'NONE', *, *, #4160, .F. ) ;
#12872=CARTESIAN_POINT ( 'NONE',  ( 11.50000000000008171, 17.32050807568872486, -17.99999999999999645 ) ) ;
#12920=ORIENTED_EDGE ( 'NONE', *, *, #24742, .T. ) ;
#12937=CARTESIAN_POINT ( 'NONE',  ( -24.99999999999999289, 60.00000000000000711, -30.00000000000000711 ) ) ;
#12966=VERTEX_POINT ( 'NONE', #12226 ) ;
#13005=CARTESIAN_POINT ( 'NONE',  ( -13.00000000000000178, -2.870178842070716726E-15, 23.00000000000000000 ) ) ;
#13025=ORIENTED_EDGE ( 'NONE', *, *, #12300, .T. ) ;
#13112=ORIENTED_EDGE ( 'NONE', *, *, #24142, .T. ) ;
#13115=DIRECTION ( 'NONE',  ( 0.000000000000000000, 0.000000000000000000, -1.000000000000000000 ) ) ;
#13146=CARTESIAN_POINT ( 'NONE',  ( -19.99999999999999289, 60.00000000000000711, -25.00000000000000000 ) ) ;
#13176=DIRECTION ( 'NONE',  ( 0.000000000000000000, -1.000000000000000000, 0.000000000000000000 ) ) ;
#13190=AXIS2_PLACEMENT_3D ( 'NONE', #5435, #19606, #10446 ) ;
#13221=CARTESIAN_POINT ( 'NONE',  ( -13.00000000000000178, -2.870178842070716726E-15, 23.00000000000000000 ) ) ;
#13233=ORIENTED_EDGE ( 'NONE', *, *, #26745, .F. ) ;
#13264=CIRCLE ( 'NONE', #112, 13.00000000000000178 ) ;
#13303=VECTOR ( 'NONE', #3050, 1000.000000000000000 ) ;
#13310=DIRECTION ( 'NONE',  ( -0.000000000000000000, 1.000000000000000000, 0.000000000000000000 ) ) ;
#13368=CARTESIAN_POINT ( 'NONE',  ( 0.000000000000000000, 0.000000000000000000, 23.00000000000000000 ) ) ;
#13454=EDGE_LOOP ( 'NONE', ( #5808, #16713, #25157, #10192, #17056, #2059, #17239, #11554 ) ) ;
#13455=FACE_OUTER_BOUND ( 'NONE', #12832, .T. ) ;
#13468=DIRECTION ( 'NONE',  ( -1.000000000000000000, 0.000000000000000000, 0.000000000000000000 ) ) ;
#13481=ORIENTED_EDGE ( 'NONE', *, *, #16792, .T. ) ;
#13496=DIRECTION ( 'NONE',  ( 5.782411586589357392E-17, -0.000000000000000000, 1.000000000000000000 ) ) ;
#13517=LINE ( 'NONE', #18096, #1775 ) ;
#13521=DIRECTION ( 'NONE',  ( 5.782411586589357392E-17, -0.000000000000000000, 1.000000000000000000 ) ) ;
#13561=ORIENTED_EDGE ( 'NONE', *, *, #15930, .F. ) ;
#13564=CARTESIAN_POINT ( 'NONE',  ( -24.99999999999998934, 60.00000000000000711, 24.99999999999998934 ) ) ;
#13648=CARTESIAN_POINT ( 'NONE',  ( -24.99999999999999289, 60.00000000000000711, -25.00000000000000000 ) ) ;
#13649=VERTEX_POINT ( 'NONE', #19976 ) ;
#13662=COLOUR_RGB ( '', 0.09019608, 0.27058824, 0.51372549) ;
#13673=LINE ( 'NONE', #16413, #26654 ) ;
#13743=VERTEX_POINT ( 'NONE', #1988 ) ;
#13765=VERTEX_POINT ( 'NONE', #30102 ) ;
#13767=ORIENTED_EDGE ( 'NONE', *, *, #4832, .T. ) ;
#13814=ORIENTED_EDGE ( 'NONE', *, *, #9968, .T. ) ;
#13826=ORIENTED_EDGE ( 'NONE', *, *, #8280, .F. ) ;
#13886=ORIENTED_EDGE ( 'NONE', *, *, #10958, .F. ) ;
#13894=VERTEX_POINT ( 'NONE', #9873 ) ;
#13909=DIRECTION ( 'NONE',  ( -1.000000000000000000, 0.000000000000000000, 0.000000000000000000 ) ) ;
#13954=DIRECTION ( 'NONE',  ( 1.000000000000000000, 0.000000000000000000, 0.000000000000000000 ) ) ;
#14056=EDGE_CURVE ( 'NONE', #10176, #27390, #14743, .T. ) ;
#14060=DIRECTION ( 'NONE',  ( -0.000000000000000000, -0.000000000000000000, 1.000000000000000000 ) ) ;
#14067=FACE_OUTER_BOUND ( 'NONE', #20989, .T. ) ;
#14074=EDGE_LOOP ( 'NONE', ( #27733, #27343, #23512, #29597 ) ) ;
#14109=ORIENTED_EDGE ( 'NONE', *, *, #28546, .T. ) ;
#14110=AXIS2_PLACEMENT_3D ( 'NONE', #15863, #8696, #29679 ) ;
#14128=VERTEX_POINT ( 'NONE', #3776 ) ;
#14213=ORIENTED_EDGE ( 'NONE', *, *, #16792, .F. ) ;
#14288=DIRECTION ( 'NONE',  ( -1.000000000000000000, 0.000000000000000000, 0.000000000000000000 ) ) ;
#14291=EDGE_LOOP ( 'NONE', ( #28463, #3535, #21819, #651 ) ) ;
#14305=ADVANCED_FACE ( 'NONE', ( #15956, #25283, #4521 ), #16256, .T. ) ;
#14363=EDGE_CURVE ( 'NONE', #24692, #3985, #13673, .T. ) ;
#14383=DIRECTION ( 'NONE',  ( -0.000000000000000000, -0.000000000000000000, -1.000000000000000000 ) ) ;
#14451=ORIENTED_EDGE ( 'NONE', *, *, #22977, .F. ) ;
#14488=CARTESIAN_POINT ( 'NONE',  ( -24.99999999999999289, 55.00000000000000711, -30.00000000000000711 ) ) ;
#14557=CARTESIAN_POINT ( 'NONE',  ( 0.000000000000000000, 55.00000000000000711, -23.00000000000000000 ) ) ;
#14592=DIRECTION ( 'NONE',  ( -0.000000000000000000, -0.000000000000000000, 1.000000000000000000 ) ) ;
#14606=EDGE_CURVE ( 'NONE', #29940, #10176, #9049, .T. ) ;
#14718=VERTEX_POINT ( 'NONE', #20201 ) ;
#14743=LINE ( 'NONE', #883, #2739 ) ;
#14793=LINE ( 'NONE', #12666, #21539 ) ;
#14806=CARTESIAN_POINT ( 'NONE',  ( 25.00000000000001066, 55.00000000000000711, 24.99999999999998579 ) ) ;
#14817=ORIENTED_EDGE ( 'NONE', *, *, #17209, .T. ) ;
#14831=DIRECTION ( 'NONE',  ( 0.000000000000000000, 0.000000000000000000, -1.000000000000000000 ) ) ;
#14888=ORIENTED_EDGE ( 'NONE', *, *, #10141, .F. ) ;
#14898=VECTOR ( 'NONE', #19134, 1000.000000000000000 ) ;
#14960=CARTESIAN_POINT ( 'NONE',  ( 19.99999999999998934, 60.00000000000000711, -30.00000000000000000 ) ) ;
#15026=AXIS2_PLACEMENT_3D ( 'NONE', #12420, #19736, #3430 ) ;
#15063=VERTEX_POINT ( 'NONE', #1921 ) ;
#15087=ADVANCED_FACE ( 'NONE', ( #18220 ), #27576, .T. ) ;
#15115=ORIENTED_EDGE ( 'NONE', *, *, #15916, .F. ) ;
#15130=EDGE_CURVE ( 'NONE', #5157, #15686, #2788, .T. ) ;
#15196=EDGE_LOOP ( 'NONE', ( #10966, #20164, #21630, #12920 ) ) ;
#15208=ADVANCED_FACE ( 'NONE', ( #7832 ), #5552, .F. ) ;
#15218=PLANE ( 'NONE',  #15560 ) ;
#15240=EDGE_CURVE ( 'NONE', #27929, #7222, #26188, .T. ) ;
#15245=ORIENTED_EDGE ( 'NONE', *, *, #2495, .T. ) ;
#15261=DIRECTION ( 'NONE',  ( -1.000000000000000000, 0.000000000000000000, 0.000000000000000000 ) ) ;
#15330=CARTESIAN_POINT ( 'NONE',  ( -19.99999999999998934, 60.00000000000000711, 24.99999999999998934 ) ) ;
#15377=ADVANCED_FACE ( 'NONE', ( #8424 ), #27084, .T. ) ;
#15424=DIRECTION ( 'NONE',  ( 0.000000000000000000, -0.000000000000000000, -1.000000000000000000 ) ) ;
#15441=DIRECTION ( 'NONE',  ( 2.207829878515935943E-16, -1.000000000000000000, 0.000000000000000000 ) ) ;
#15460=CARTESIAN_POINT ( 'NONE',  ( 0.000000000000000000, 55.00000000000000711, 0.000000000000000000 ) ) ;
#15466=ORIENTED_EDGE ( 'NONE', *, *, #26745, .T. ) ;
#15522=EDGE_CURVE ( 'NONE', #15063, #17767, #17429, .T. ) ;
#15560=AXIS2_PLACEMENT_3D ( 'NONE', #12937, #1209, #3497 ) ;
#15574=ORIENTED_EDGE ( 'NONE', *, *, #8015, .F. ) ;
#15613=FACE_BOUND ( 'NONE', #12773, .T. ) ;
#15686=VERTEX_POINT ( 'NONE', #29859 ) ;
#15722=EDGE_CURVE ( 'NONE', #13765, #13649, #30152, .T. ) ;
#15780=AXIS2_PLACEMENT_3D ( 'NONE', #5783, #19506, #5480 ) ;
#15798=CARTESIAN_POINT ( 'NONE',  ( 8.500000000000088818, 17.32050807568872486, -17.99999999999999645 ) ) ;
#15825=DIRECTION ( 'NONE',  ( 1.000000000000000000, 0.000000000000000000, 0.000000000000000000 ) ) ;
#15863=CARTESIAN_POINT ( 'NONE',  ( 0.000000000000000000, 0.000000000000000000, -18.00000000000000000 ) ) ;
#15878=VERTEX_POINT ( 'NONE', #3670 ) ;
#15895=CARTESIAN_POINT ( 'NONE',  ( 20.00000000000001066, 60.00000000000000711, 24.99999999999998579 ) ) ;
#15907=CARTESIAN_POINT ( 'NONE',  ( 0.000000000000000000, 0.000000000000000000, 23.00000000000000000 ) ) ;
#15916=EDGE_CURVE ( 'NONE', #18267, #25189, #14793, .T. ) ;
#15930=EDGE_CURVE ( 'NONE', #29592, #19798, #13264, .T. ) ;
#15956=FACE_BOUND ( 'NONE', #12151, .T. ) ;
#15963=ORIENTED_EDGE ( 'NONE', *, *, #1239, .T. ) ;
#16031=DIRECTION ( 'NONE',  ( -6.938893903907227392E-16, 0.000000000000000000, -1.000000000000000000 ) ) ;
#16057=PLANE ( 'NONE',  #827 ) ;
#16104=CARTESIAN_POINT ( 'NONE',  ( 5.000000000000000000, 6.123233995736766282E-16, 18.00000000000000000 ) ) ;
#16138=DIRECTION ( 'NONE',  ( 0.000000000000000000, -1.000000000000000000, 0.000000000000000000 ) ) ;
#16197=DIRECTION ( 'NONE',  ( -2.207829878515935943E-16, 1.000000000000000000, 0.000000000000000000 ) ) ;
#16208=AXIS2_PLACEMENT_3D ( 'NONE', #23087, #8877, #9171 ) ;
#16256=PLANE ( 'NONE',  #19303 ) ;
#16283=CIRCLE ( 'NONE', #7050, 1.499999999999996225 ) ;
#16289=LINE ( 'NONE', #433, #11707 ) ;
#16307=ORIENTED_EDGE ( 'NONE', *, *, #1239, .F. ) ;
#16326=EDGE_LOOP ( 'NONE', ( #25587, #18314 ) ) ;
#16345=( GEOMETRIC_REPRESENTATION_CONTEXT ( 3 ) GLOBAL_UNCERTAINTY_ASSIGNED_CONTEXT ( ( #23234 ) ) GLOBAL_UNIT_ASSIGNED_CONTEXT ( ( #2237, #243, #23277 ) ) REPRESENTATION_CONTEXT ( 'NONE', 'WORKASPACE' ) );
#16389=LINE ( 'NONE', #4500, #4393 ) ;
#16413=CARTESIAN_POINT ( 'NONE',  ( -24.99999999999998934, 60.00000000000000711, 29.99999999999999289 ) ) ;
#16442=EDGE_CURVE ( 'NONE', #29543, #14718, #29425, .T. ) ;
#16447=DIRECTION ( 'NONE',  ( 1.000000000000000000, 0.000000000000000000, 0.000000000000000000 ) ) ;
#16450=ORIENTED_EDGE ( 'NONE', *, *, #9968, .F. ) ;
#16545=LINE ( 'NONE', #18988, #3527 ) ;
#16547=LINE ( 'NONE', #26175, #23571 ) ;
#16602=CARTESIAN_POINT ( 'NONE',  ( 10.00000000000008527, 17.32050807568872486, -30.00000000000000711 ) ) ;
#16620=CARTESIAN_POINT ( 'NONE',  ( -5.000000000000000000, 0.000000000000000000, -18.00000000000000000 ) ) ;
#16665=LINE ( 'NONE', #4914, #27572 ) ;
#16668=ORIENTED_EDGE ( 'NONE', *, *, #5713, .F. ) ;
#16700=APPLICATION_CONTEXT ( 'automotive_design' ) ;
#16713=ORIENTED_EDGE ( 'NONE', *, *, #24489, .T. ) ;
#16737=DIRECTION ( 'NONE',  ( 0.000000000000000000, -1.000000000000000000, 0.000000000000000000 ) ) ;
#16792=EDGE_CURVE ( 'NONE', #5157, #29543, #12402, .T. ) ;
#16824=EDGE_CURVE ( 'NONE', #13894, #30129, #2586, .T. ) ;
#16849=AXIS2_PLACEMENT_3D ( 'NONE', #12162, #14592, #14288 ) ;
#16865=DIRECTION ( 'NONE',  ( 1.000000000000000000, 0.000000000000000000, -5.782411586589357392E-17 ) ) ;
#16913=DIRECTION ( 'NONE',  ( 1.000000000000000000, 0.000000000000000000, 0.000000000000000000 ) ) ;
#17003=EDGE_CURVE ( 'NONE', #10176, #28903, #26091, .T. ) ;
#17007=CIRCLE ( 'NONE', #22880, 12.50000000000000000 ) ;
#17016=CARTESIAN_POINT ( 'NONE',  ( 6.938893903907228378E-15, 60.00000000000000711, -1.040834085586084257E-14 ) ) ;
#17023=FACE_OUTER_BOUND ( 'NONE', #5989, .T. ) ;
#17033=LINE ( 'NONE', #10304, #12820 ) ;
#17056=ORIENTED_EDGE ( 'NONE', *, *, #5713, .T. ) ;
#17090=CYLINDRICAL_SURFACE ( 'NONE', #23271, 5.000000000000000000 ) ;
#17091=VERTEX_POINT ( 'NONE', #22409 ) ;
#17140=CARTESIAN_POINT ( 'NONE',  ( 6.938893903907228378E-15, 60.00000000000000711, -1.040834085586084257E-14 ) ) ;
#17150=DIRECTION ( 'NONE',  ( -2.207829878515935943E-16, -1.000000000000000000, -0.000000000000000000 ) ) ;
#17160=FACE_BOUND ( 'NONE', #19248, .T. ) ;
#17189=DIRECTION ( 'NONE',  ( -0.000000000000000000, 1.000000000000000000, 0.000000000000000000 ) ) ;
#17209=EDGE_CURVE ( 'NONE', #30129, #27390, #1514, .T. ) ;
#17215=EDGE_CURVE ( 'NONE', #17767, #846, #22568, .T. ) ;
#17239=ORIENTED_EDGE ( 'NONE', *, *, #3645, .T. ) ;
#17257=CYLINDRICAL_SURFACE ( 'NONE', #22354, 5.000000000000000888 ) ;
#17270=VECTOR ( 'NONE', #27857, 1000.000000000000000 ) ;
#17306=FACE_OUTER_BOUND ( 'NONE', #17722, .T. ) ;
#17320=( LENGTH_UNIT ( ) NAMED_UNIT ( * ) SI_UNIT ( .MILLI., .METRE. ) );
#17326=AXIS2_PLACEMENT_3D ( 'NONE', #18236, #27594, #17930 ) ;
#17337=DIRECTION ( 'NONE',  ( 2.207829878515935943E-16, 1.000000000000000000, 0.000000000000000000 ) ) ;
#17429=LINE ( 'NONE', #30003, #1103 ) ;
#17436=CARTESIAN_POINT ( 'NONE',  ( 6.938893903907228378E-15, 60.00000000000000711, -1.040834085586084257E-14 ) ) ;
#17458=ORIENTED_EDGE ( 'NONE', *, *, #7943, .T. ) ;
#17517=EDGE_CURVE ( 'NONE', #27580, #10204, #17033, .T. ) ;
#17580=DIRECTION ( 'NONE',  ( -1.000000000000000000, -2.207829878515935943E-16, 0.000000000000000000 ) ) ;
#17618=SURFACE_STYLE_USAGE ( .BOTH. , #10147 ) ;
#17704=PRODUCT_DEFINITION_CONTEXT ( 'detailed design', #16700, 'design' ) ;
#17722=EDGE_LOOP ( 'NONE', ( #15963, #24658, #22585, #26773 ) ) ;
#17767=VERTEX_POINT ( 'NONE', #22069 ) ;
#17781=FACE_OUTER_BOUND ( 'NONE', #3550, .T. ) ;
#17819=STYLED_ITEM ( 'NONE', ( #20980 ), #21231 ) ;
#17836=ORIENTED_EDGE ( 'NONE', *, *, #18578, .T. ) ;
#17853=EDGE_CURVE ( 'NONE', #24692, #13894, #1928, .T. ) ;
#17887=FACE_BOUND ( 'NONE', #16326, .T. ) ;
#17914=EDGE_CURVE ( 'NONE', #7269, #653, #29904, .T. ) ;
#17930=DIRECTION ( 'NONE',  ( 0.000000000000000000, 0.000000000000000000, -1.000000000000000000 ) ) ;
#18050=DIRECTION ( 'NONE',  ( 0.000000000000000000, 0.000000000000000000, -1.000000000000000000 ) ) ;
#18096=CARTESIAN_POINT ( 'NONE',  ( 0.000000000000000000, 55.00000000000000711, 23.00000000000000000 ) ) ;
#18133=EDGE_CURVE ( 'NONE', #8000, #5008, #16547, .T. ) ;
#18196=CARTESIAN_POINT ( 'NONE',  ( 6.938893903907228378E-15, 60.00000000000000711, -12.50000000000001066 ) ) ;
#18220=FACE_OUTER_BOUND ( 'NONE', #27478, .T. ) ;
#18236=CARTESIAN_POINT ( 'NONE',  ( -19.99999999999998934, 60.00000000000000711, 24.99999999999998934 ) ) ;
#18267=VERTEX_POINT ( 'NONE', #27255 ) ;
#18307=EDGE_LOOP ( 'NONE', ( #5591, #14451 ) ) ;
#18314=ORIENTED_EDGE ( 'NONE', *, *, #8280, .T. ) ;
#18351=FACE_BOUND ( 'NONE', #14074, .T. ) ;
#18392=FILL_AREA_STYLE ('',( #20823 ) ) ;
#18409=ORIENTED_EDGE ( 'NONE', *, *, #17003, .F. ) ;
#18417=VECTOR ( 'NONE', #12358, 1000.000000000000000 ) ;
#18439=CIRCLE ( 'NONE', #21353, 5.000000000000000888 ) ;
#18463=AXIS2_PLACEMENT_3D ( 'NONE', #4431, #20594, #23192 ) ;
#18500=AXIS2_PLACEMENT_3D ( 'NONE', #9249, #30090, #9100 ) ;
#18534=CARTESIAN_POINT ( 'NONE',  ( 11.50000000000008171, 17.32050807568872486, -30.00000000000000711 ) ) ;
#18553=DIRECTION ( 'NONE',  ( 1.000000000000000000, 0.000000000000000000, 0.000000000000000000 ) ) ;
#18578=EDGE_CURVE ( 'NONE', #22249, #20836, #25056, .T. ) ;
#18617=VERTEX_POINT ( 'NONE', #8054 ) ;
#18621=VECTOR ( 'NONE', #16197, 1000.000000000000000 ) ;
#18728=EDGE_CURVE ( 'NONE', #17091, #29924, #28002, .T. ) ;
#18780=LINE ( 'NONE', #14488, #20806 ) ;
#18809=VECTOR ( 'NONE', #3978, 1000.000000000000000 ) ;
#18841=ORIENTED_EDGE ( 'NONE', *, *, #15130, .F. ) ;
#18889=CYLINDRICAL_SURFACE ( 'NONE', #23423, 1.499999999999996225 ) ;
#18988=CARTESIAN_POINT ( 'NONE',  ( 20.00000000000000711, 60.00000000000000711, 29.99999999999998579 ) ) ;
#19058=CARTESIAN_POINT ( 'NONE',  ( 25.00000000000000000, 60.00000000000000711, -24.99999999999999289 ) ) ;
#19134=DIRECTION ( 'NONE',  ( 2.207829878515935943E-16, 1.000000000000000000, 0.000000000000000000 ) ) ;
#19197=AXIS2_PLACEMENT_3D ( 'NONE', #22570, #10950, #15825 ) ;
#19230=CARTESIAN_POINT ( 'NONE',  ( -13.00000000000000178, -2.870178842070716726E-15, -23.00000000000000000 ) ) ;
#19248=EDGE_LOOP ( 'NONE', ( #14109, #28277 ) ) ;
#19268=DIRECTION ( 'NONE',  ( 0.000000000000000000, 0.000000000000000000, -1.000000000000000000 ) ) ;
#19296=CYLINDRICAL_SURFACE ( 'NONE', #27371, 12.50000000000000000 ) ;
#19303=AXIS2_PLACEMENT_3D ( 'NONE', #27464, #25569, #18553 ) ;
#19376=ORIENTED_EDGE ( 'NONE', *, *, #17853, .F. ) ;
#19394=DIRECTION ( 'NONE',  ( 1.000000000000000000, 0.000000000000000000, 0.000000000000000000 ) ) ;
#19506=DIRECTION ( 'NONE',  ( -0.000000000000000000, 0.000000000000000000, 1.000000000000000000 ) ) ;
#19519=MECHANICAL_DESIGN_GEOMETRIC_PRESENTATION_REPRESENTATION('',(#20979),#5883);
#19576=ORIENTED_EDGE ( 'NONE', *, *, #24665, .F. ) ;
#19581=PLANE ( 'NONE',  #8615 ) ;
#19606=DIRECTION ( 'NONE',  ( 0.000000000000000000, 0.000000000000000000, 1.000000000000000000 ) ) ;
#19642=DIRECTION ( 'NONE',  ( -0.000000000000000000, -0.000000000000000000, 1.000000000000000000 ) ) ;
#19654=VECTOR ( 'NONE', #11654, 1000.000000000000000 ) ;
#19662=ORIENTED_EDGE ( 'NONE', *, *, #8869, .T. ) ;
#19727=CARTESIAN_POINT ( 'NONE',  ( 13.00000000000000178, -2.870178842070716726E-15, -23.00000000000000000 ) ) ;
#19736=DIRECTION ( 'NONE',  ( 0.000000000000000000, 0.000000000000000000, -1.000000000000000000 ) ) ;
#19739=AXIS2_PLACEMENT_3D ( 'NONE', #24291, #10386, #15261 ) ;
#19798=VERTEX_POINT ( 'NONE', #26481 ) ;
#19822=ORIENTED_EDGE ( 'NONE', *, *, #14363, .F. ) ;
#19851=ORIENTED_EDGE ( 'NONE', *, *, #15240, .F. ) ;
#19858=ORIENTED_EDGE ( 'NONE', *, *, #14606, .F. ) ;
#19876=DIRECTION ( 'NONE',  ( 1.000000000000000000, 0.000000000000000000, 0.000000000000000000 ) ) ;
#19892=CARTESIAN_POINT ( 'NONE',  ( 25.00000000000001066, 60.00000000000000711, 29.99999999999998579 ) ) ;
#19954=DIRECTION ( 'NONE',  ( 0.000000000000000000, -0.000000000000000000, -1.000000000000000000 ) ) ;
#19976=CARTESIAN_POINT ( 'NONE',  ( -13.00000000000001243, 55.00000000000000711, -23.00000000000000000 ) ) ;
#20072=CIRCLE ( 'NONE', #7894, 5.000000000000000000 ) ;
#20097=EDGE_LOOP ( 'NONE', ( #16307, #24027 ) ) ;
#20110=CARTESIAN_POINT ( 'NONE',  ( -19.99999999999999289, 60.00000000000000711, -30.00000000000000711 ) ) ;
#20147=ORIENTED_EDGE ( 'NONE', *, *, #16442, .F. ) ;
#20164=ORIENTED_EDGE ( 'NONE', *, *, #26323, .F. ) ;
#20201=CARTESIAN_POINT ( 'NONE',  ( -5.000000000000000000, 0.000000000000000000, 18.00000000000000000 ) ) ;
#20237=EDGE_CURVE ( 'NONE', #29592, #15878, #16665, .T. ) ;
#20254=VERTEX_POINT ( 'NONE', #26138 ) ;
#20319=AXIS2_PLACEMENT_3D ( 'NONE', #9942, #22152, #26600 ) ;
#20327=LINE ( 'NONE', #8579, #12028 ) ;
#20356=DIRECTION ( 'NONE',  ( 0.000000000000000000, 0.000000000000000000, -1.000000000000000000 ) ) ;
#20365=ADVANCED_FACE ( 'NONE', ( #7365, #2640 ), #351, .T. ) ;
#20434=DIRECTION ( 'NONE',  ( 1.000000000000000000, 0.000000000000000000, 0.000000000000000000 ) ) ;
#20447=ORIENTED_EDGE ( 'NONE', *, *, #16442, .T. ) ;
#20455=CARTESIAN_POINT ( 'NONE',  ( 0.000000000000000000, 0.000000000000000000, 23.00000000000000000 ) ) ;
#20456=VECTOR ( 'NONE', #27557, 1000.000000000000000 ) ;
#20575=ORIENTED_EDGE ( 'NONE', *, *, #303, .F. ) ;
#20582=ORIENTED_EDGE ( 'NONE', *, *, #17215, .T. ) ;
#20594=DIRECTION ( 'NONE',  ( -0.000000000000000000, 0.000000000000000000, 1.000000000000000000 ) ) ;
#20621=EDGE_CURVE ( 'NONE', #7269, #8000, #4649, .T. ) ;
#20678=DIRECTION ( 'NONE',  ( -0.000000000000000000, -0.000000000000000000, -1.000000000000000000 ) ) ;
#20769=CARTESIAN_POINT ( 'NONE',  ( -24.99999999999998934, 60.00000000000000711, 29.99999999999999289 ) ) ;
#20773=AXIS2_PLACEMENT_3D ( 'NONE', #21106, #21560, #7520 ) ;
#20803=ORIENTED_EDGE ( 'NONE', *, *, #8034, .T. ) ;
#20806=VECTOR ( 'NONE', #23513, 1000.000000000000000 ) ;
#20823=FILL_AREA_STYLE_COLOUR ( '', #3236 ) ;
#20830=FACE_OUTER_BOUND ( 'NONE', #6126, .T. ) ;
#20836=VERTEX_POINT ( 'NONE', #5908 ) ;
#20840=ORIENTED_EDGE ( 'NONE', *, *, #3989, .F. ) ;
#20902=ORIENTED_EDGE ( 'NONE', *, *, #2495, .F. ) ;
#20979=STYLED_ITEM ( 'NONE', ( #21906 ), #29596 ) ;
#20980=PRESENTATION_STYLE_ASSIGNMENT (( #6959 ) ) ;
#20989=EDGE_LOOP ( 'NONE', ( #3687, #26896, #26021, #19376 ) ) ;
#21010=EDGE_LOOP ( 'NONE', ( #1305, #24019, #28489, #9483 ) ) ;
#21046=CARTESIAN_POINT ( 'NONE',  ( 0.000000000000000000, 0.000000000000000000, 18.00000000000000000 ) ) ;
#21055=ORIENTED_EDGE ( 'NONE', *, *, #28844, .F. ) ;
#21073=ORIENTED_EDGE ( 'NONE', *, *, #7733, .F. ) ;
#21084=AXIS2_PLACEMENT_3D ( 'NONE', #10644, #19954, #26543 ) ;
#21106=CARTESIAN_POINT ( 'NONE',  ( 0.000000000000000000, 0.000000000000000000, -23.00000000000000000 ) ) ;
#21129=ADVANCED_FACE ( 'NONE', ( #17781 ), #27141, .T. ) ;
#21193=FACE_BOUND ( 'NONE', #24930, .T. ) ;
#21231=MANIFOLD_SOLID_BREP ( 'Cut-Extrude1', #8718 ) ;
#21353=AXIS2_PLACEMENT_3D ( 'NONE', #25181, #27648, #2147 ) ;
#21386=AXIS2_PLACEMENT_3D ( 'NONE', #11011, #19642, #3047 ) ;
#21390=AXIS2_PLACEMENT_3D ( 'NONE', #9370, #89, #7259 ) ;
#21523=DIRECTION ( 'NONE',  ( -0.000000000000000000, -0.000000000000000000, -1.000000000000000000 ) ) ;
#21539=VECTOR ( 'NONE', #24132, 1000.000000000000000 ) ;
#21542=CARTESIAN_POINT ( 'NONE',  ( 20.00000000000001066, 60.00000000000000711, 24.99999999999998579 ) ) ;
#21549=ORIENTED_EDGE ( 'NONE', *, *, #303, .T. ) ;
#21560=DIRECTION ( 'NONE',  ( -0.000000000000000000, -0.000000000000000000, 1.000000000000000000 ) ) ;
#21561=EDGE_CURVE ( 'NONE', #15878, #23534, #1601, .T. ) ;
#21598=ORIENTED_EDGE ( 'NONE', *, *, #467, .T. ) ;
#21630=ORIENTED_EDGE ( 'NONE', *, *, #2218, .F. ) ;
#21640=DIRECTION ( 'NONE',  ( -0.000000000000000000, -0.000000000000000000, -1.000000000000000000 ) ) ;
#21660=FACE_OUTER_BOUND ( 'NONE', #27376, .T. ) ;
#21738=FACE_BOUND ( 'NONE', #18307, .T. ) ;
#21756=( NAMED_UNIT ( * ) SI_UNIT ( $, .STERADIAN. ) SOLID_ANGLE_UNIT ( ) );
#21767=EDGE_CURVE ( 'NONE', #7222, #17091, #22747, .T. ) ;
#21819=ORIENTED_EDGE ( 'NONE', *, *, #3645, .F. ) ;
#21835=CIRCLE ( 'NONE', #24285, 5.000000000000000888 ) ;
#21906=PRESENTATION_STYLE_ASSIGNMENT (( #17618 ) ) ;
#21960=ORIENTED_EDGE ( 'NONE', *, *, #4160, .T. ) ;
#22019=PRODUCT ( 'base plate', 'base plate', '', ( #3232 ) ) ;
#22069=CARTESIAN_POINT ( 'NONE',  ( -19.99999999999998934, 55.00000000000000711, 29.99999999999999289 ) ) ;
#22152=DIRECTION ( 'NONE',  ( -0.000000000000000000, -0.000000000000000000, 1.000000000000000000 ) ) ;
#22166=ADVANCED_FACE ( 'NONE', ( #15613, #17887, #6765, #18351 ), #16057, .T. ) ;
#22188=CARTESIAN_POINT ( 'NONE',  ( -24.99999999999998934, 60.00000000000000711, 29.99999999999999289 ) ) ;
#22224=DIRECTION ( 'NONE',  ( 0.000000000000000000, 0.000000000000000000, -1.000000000000000000 ) ) ;
#22249=VERTEX_POINT ( 'NONE', #28007 ) ;
#22269=DIRECTION ( 'NONE',  ( 1.734723475976807587E-16, 0.000000000000000000, 1.000000000000000000 ) ) ;
#22275=VERTEX_POINT ( 'NONE', #28462 ) ;
#22276=VECTOR ( 'NONE', #3815, 1000.000000000000000 ) ;
#22287=CARTESIAN_POINT ( 'NONE',  ( 5.000000000000000000, -6.123233995736766282E-16, -23.00000000000000000 ) ) ;
#22314=ORIENTED_EDGE ( 'NONE', *, *, #3862, .F. ) ;
#22326=VECTOR ( 'NONE', #11761, 1000.000000000000000 ) ;
#22331=DIRECTION ( 'NONE',  ( 0.000000000000000000, 1.000000000000000000, 0.000000000000000000 ) ) ;
#22354=AXIS2_PLACEMENT_3D ( 'NONE', #21542, #643, #26587 ) ;
#22364=( NAMED_UNIT ( * ) SI_UNIT ( $, .STERADIAN. ) SOLID_ANGLE_UNIT ( ) );
#22380=CYLINDRICAL_SURFACE ( 'NONE', #27808, 1.499999999999996225 ) ;
#22398=CIRCLE ( 'NONE', #9209, 12.50000000000000000 ) ;
#22409=CARTESIAN_POINT ( 'NONE',  ( 5.000000000000000000, -6.123233995736766282E-16, -18.00000000000000000 ) ) ;
#22432=FACE_OUTER_BOUND ( 'NONE', #14291, .T. ) ;
#22489=DIRECTION ( 'NONE',  ( -0.000000000000000000, -0.000000000000000000, -1.000000000000000000 ) ) ;
#22542=CARTESIAN_POINT ( 'NONE',  ( 5.000000000000000000, 6.123233995736766282E-16, 23.00000000000000000 ) ) ;
#22543=LINE ( 'NONE', #24374, #26627 ) ;
#22568=LINE ( 'NONE', #1666, #7942 ) ;
#22570=CARTESIAN_POINT ( 'NONE',  ( 0.000000000000000000, 0.000000000000000000, -18.00000000000000000 ) ) ;
#22585=ORIENTED_EDGE ( 'NONE', *, *, #1665, .F. ) ;
#22633=DIRECTION ( 'NONE',  ( 2.081668171172168119E-15, 0.000000000000000000, -1.000000000000000000 ) ) ;
#22692=CYLINDRICAL_SURFACE ( 'NONE', #22722, 5.000000000000000000 ) ;
#22722=AXIS2_PLACEMENT_3D ( 'NONE', #13368, #20678, #11231 ) ;
#22747=LINE ( 'NONE', #22287, #18809 ) ;
#22784=DIRECTION ( 'NONE',  ( -1.387778780781445676E-16, 0.000000000000000000, -1.000000000000000000 ) ) ;
#22806=VERTEX_POINT ( 'NONE', #3841 ) ;
#22846=EDGE_LOOP ( 'NONE', ( #30130, #9853 ) ) ;
#22880=AXIS2_PLACEMENT_3D ( 'NONE', #17436, #22331, #8575 ) ;
#22973=CIRCLE ( 'NONE', #4918, 5.000000000000000888 ) ;
#22977=EDGE_CURVE ( 'NONE', #5008, #653, #29139, .T. ) ;
#23047=CIRCLE ( 'NONE', #3543, 5.000000000000000888 ) ;
#23087=CARTESIAN_POINT ( 'NONE',  ( 6.938893903907228378E-15, 55.00000000000000711, -1.040834085586084257E-14 ) ) ;
#23192=DIRECTION ( 'NONE',  ( 1.000000000000000000, 0.000000000000000000, 0.000000000000000000 ) ) ;
#23204=ADVANCED_FACE ( 'NONE', ( #20830 ), #22692, .F. ) ;
#23210=EDGE_CURVE ( 'NONE', #15878, #4416, #13517, .T. ) ;
#23220=FACE_OUTER_BOUND ( 'NONE', #12706, .T. ) ;
#23227=AXIS2_PLACEMENT_3D ( 'NONE', #7241, #26313, #28626 ) ;
#23234=UNCERTAINTY_MEASURE_WITH_UNIT (LENGTH_MEASURE( 1.000000000000000082E-05 ), #2237, 'distance_accuracy_value', 'NONE');
#23268=DIRECTION ( 'NONE',  ( 0.000000000000000000, -1.000000000000000000, 0.000000000000000000 ) ) ;
#23271=AXIS2_PLACEMENT_3D ( 'NONE', #5798, #28575, #26415 ) ;
#23277=( NAMED_UNIT ( * ) SI_UNIT ( $, .STERADIAN. ) SOLID_ANGLE_UNIT ( ) );
#23312=FACE_BOUND ( 'NONE', #20097, .T. ) ;
#23369=DIRECTION ( 'NONE',  ( 2.207829878515935943E-16, -1.000000000000000000, 0.000000000000000000 ) ) ;
#23401=LINE ( 'NONE', #2518, #6159 ) ;
#23423=AXIS2_PLACEMENT_3D ( 'NONE', #16602, #28542, #16447 ) ;
#23426=AXIS2_PLACEMENT_3D ( 'NONE', #23549, #361, #2054 ) ;
#23468=PLANE ( 'NONE',  #6378 ) ;
#23497=EDGE_LOOP ( 'NONE', ( #24736, #29816, #11406, #13826 ) ) ;
#23512=ORIENTED_EDGE ( 'NONE', *, *, #23210, .T. ) ;
#23513=DIRECTION ( 'NONE',  ( -1.000000000000000000, -0.000000000000000000, -1.387778780781445922E-16 ) ) ;
#23524=LINE ( 'NONE', #5205, #22326 ) ;
#23534=VERTEX_POINT ( 'NONE', #94 ) ;
#23549=CARTESIAN_POINT ( 'NONE',  ( -19.99999999999999289, 60.00000000000000711, -25.00000000000000000 ) ) ;
#23571=VECTOR ( 'NONE', #23572, 1000.000000000000000 ) ;
#23572=DIRECTION ( 'NONE',  ( 0.000000000000000000, 0.000000000000000000, 1.000000000000000000 ) ) ;
#23617=CARTESIAN_POINT ( 'NONE',  ( 0.000000000000000000, 60.00000000000000711, 0.000000000000000000 ) ) ;
#23871=ORIENTED_EDGE ( 'NONE', *, *, #8034, .F. ) ;
#23883=CARTESIAN_POINT ( 'NONE',  ( 5.000000000000000000, 6.123233995736766282E-16, 23.00000000000000000 ) ) ;
#23904=DIRECTION ( 'NONE',  ( 1.000000000000000000, 0.000000000000000000, 0.000000000000000000 ) ) ;
#23936=CARTESIAN_POINT ( 'NONE',  ( -19.99999999999998934, 55.00000000000000711, 24.99999999999998934 ) ) ;
#23961=CARTESIAN_POINT ( 'NONE',  ( 20.00000000000000355, 60.00000000000000711, -30.00000000000000000 ) ) ;
#24019=ORIENTED_EDGE ( 'NONE', *, *, #8951, .F. ) ;
#24022=ADVANCED_FACE ( 'NONE', ( #28614 ), #2364, .T. ) ;
#24027=ORIENTED_EDGE ( 'NONE', *, *, #951, .F. ) ;
#24132=DIRECTION ( 'NONE',  ( 2.207829878515935943E-16, 1.000000000000000000, 0.000000000000000000 ) ) ;
#24142=EDGE_CURVE ( 'NONE', #14128, #22275, #23401, .T. ) ;
#24148=SHAPE_REPRESENTATION ( 'base plate', ( #13190 ), #3942 ) ;
#24218=ORIENTED_EDGE ( 'NONE', *, *, #23210, .F. ) ;
#24285=AXIS2_PLACEMENT_3D ( 'NONE', #15330, #17189, #8171 ) ;
#24291=CARTESIAN_POINT ( 'NONE',  ( 10.00000000000008527, 17.32050807568872486, -23.00000000000000000 ) ) ;
#24374=CARTESIAN_POINT ( 'NONE',  ( 13.00000000000000178, -2.870178842070716726E-15, 18.00000000000000000 ) ) ;
#24399=DIRECTION ( 'NONE',  ( 0.000000000000000000, 1.000000000000000000, 0.000000000000000000 ) ) ;
#24489=EDGE_CURVE ( 'NONE', #27390, #24692, #8101, .T. ) ;
#24509=CIRCLE ( 'NONE', #2102, 5.000000000000000000 ) ;
#24533=ORIENTED_EDGE ( 'NONE', *, *, #24142, .F. ) ;
#24539=ORIENTED_EDGE ( 'NONE', *, *, #15916, .T. ) ;
#24551=ORIENTED_EDGE ( 'NONE', *, *, #17003, .T. ) ;
#24658=ORIENTED_EDGE ( 'NONE', *, *, #775, .T. ) ;
#24665=EDGE_CURVE ( 'NONE', #28903, #30129, #18780, .T. ) ;
#24667=ORIENTED_EDGE ( 'NONE', *, *, #17215, .F. ) ;
#24674=FACE_OUTER_BOUND ( 'NONE', #6572, .T. ) ;
#24692=VERTEX_POINT ( 'NONE', #4743 ) ;
#24736=ORIENTED_EDGE ( 'NONE', *, *, #775, .F. ) ;
#24742=EDGE_CURVE ( 'NONE', #19798, #20836, #12809, .T. ) ;
#24778=LINE ( 'NONE', #29091, #4003 ) ;
#24824=CARTESIAN_POINT ( 'NONE',  ( 6.938893903907228378E-15, 55.00000000000000711, -12.50000000000001066 ) ) ;
#24930=EDGE_LOOP ( 'NONE', ( #9745, #20147 ) ) ;
#25004=CARTESIAN_POINT ( 'NONE',  ( -19.99999999999999645, 60.00000000000000711, -30.00000000000000711 ) ) ;
#25043=EDGE_CURVE ( 'NONE', #27247, #3985, #1684, .T. ) ;
#25056=CIRCLE ( 'NONE', #15780, 13.00000000000000178 ) ;
#25157=ORIENTED_EDGE ( 'NONE', *, *, #14363, .T. ) ;
#25171=CARTESIAN_POINT ( 'NONE',  ( 25.00000000000001066, 60.00000000000000711, 29.99999999999998579 ) ) ;
#25181=CARTESIAN_POINT ( 'NONE',  ( 20.00000000000001066, 55.00000000000000711, 24.99999999999998579 ) ) ;
#25183=CARTESIAN_POINT ( 'NONE',  ( 0.000000000000000000, 0.000000000000000000, 23.00000000000000000 ) ) ;
#25184=AXIS2_PLACEMENT_3D ( 'NONE', #13146, #6739, #16031 ) ;
#25189=VERTEX_POINT ( 'NONE', #12013 ) ;
#25283=FACE_OUTER_BOUND ( 'NONE', #29979, .T. ) ;
#25333=DIRECTION ( 'NONE',  ( -0.000000000000000000, 0.000000000000000000, 1.000000000000000000 ) ) ;
#25365=VECTOR ( 'NONE', #12275, 1000.000000000000000 ) ;
#25378=UNCERTAINTY_MEASURE_WITH_UNIT (LENGTH_MEASURE( 1.000000000000000082E-05 ), #17320, 'distance_accuracy_value', 'NONE');
#25440=DIRECTION ( 'NONE',  ( 0.000000000000000000, -1.000000000000000000, -0.000000000000000000 ) ) ;
#25518=EDGE_LOOP ( 'NONE', ( #21598, #26343, #7717, #29198 ) ) ;
#25532=CYLINDRICAL_SURFACE ( 'NONE', #23426, 5.000000000000000888 ) ;
#25560=FACE_OUTER_BOUND ( 'NONE', #15196, .T. ) ;
#25569=DIRECTION ( 'NONE',  ( 0.000000000000000000, 0.000000000000000000, -1.000000000000000000 ) ) ;
#25587=ORIENTED_EDGE ( 'NONE', *, *, #1665, .T. ) ;
#25606=ORIENTED_EDGE ( 'NONE', *, *, #12719, .F. ) ;
#25681=AXIS2_PLACEMENT_3D ( 'NONE', #10870, #22489, #27257 ) ;
#25685=ORIENTED_EDGE ( 'NONE', *, *, #24665, .T. ) ;
#25690=ORIENTED_EDGE ( 'NONE', *, *, #21767, .T. ) ;
#25718=AXIS2_PLACEMENT_3D ( 'NONE', #25171, #8376, #22269 ) ;
#25825=ORIENTED_EDGE ( 'NONE', *, *, #26824, .T. ) ;
#25845=ORIENTED_EDGE ( 'NONE', *, *, #20621, .T. ) ;
#25861=DIRECTION ( 'NONE',  ( 1.000000000000000000, 0.000000000000000000, 0.000000000000000000 ) ) ;
#26021=ORIENTED_EDGE ( 'NONE', *, *, #16824, .F. ) ;
#26091=LINE ( 'NONE', #23961, #13303 ) ;
#26138=CARTESIAN_POINT ( 'NONE',  ( 8.469702402841419307E-15, 60.00000000000000711, 12.49999999999999112 ) ) ;
#26175=CARTESIAN_POINT ( 'NONE',  ( 8.500000000000088818, 17.32050807568872486, -30.00000000000000711 ) ) ;
#26188=CIRCLE ( 'NONE', #27665, 5.000000000000000000 ) ;
#26313=DIRECTION ( 'NONE',  ( 0.000000000000000000, -0.000000000000000000, -1.000000000000000000 ) ) ;
#26323=EDGE_CURVE ( 'NONE', #4416, #6999, #23524, .T. ) ;
#26343=ORIENTED_EDGE ( 'NONE', *, *, #1837, .T. ) ;
#26364=ADVANCED_FACE ( 'NONE', ( #23220 ), #9917, .T. ) ;
#26367=EDGE_LOOP ( 'NONE', ( #19851, #23871 ) ) ;
#26415=DIRECTION ( 'NONE',  ( -1.000000000000000000, 0.000000000000000000, 0.000000000000000000 ) ) ;
#26424=CARTESIAN_POINT ( 'NONE',  ( 25.00000000000001066, 55.00000000000000711, 29.99999999999998579 ) ) ;
#26440=FACE_OUTER_BOUND ( 'NONE', #26696, .T. ) ;
#26479=LINE ( 'NONE', #2988, #14898 ) ;
#26481=CARTESIAN_POINT ( 'NONE',  ( 13.00000000000000178, -2.870178842070716726E-15, 23.00000000000000000 ) ) ;
#26505=FILL_AREA_STYLE ('',( #8313 ) ) ;
#26543=DIRECTION ( 'NONE',  ( 1.000000000000000000, 0.000000000000000000, 0.000000000000000000 ) ) ;
#26563=EDGE_CURVE ( 'NONE', #10204, #22806, #28745, .T. ) ;
#26579=SHAPE_DEFINITION_REPRESENTATION ( #12487, #24148 ) ;
#26587=DIRECTION ( 'NONE',  ( 0.000000000000000000, 0.000000000000000000, -1.000000000000000000 ) ) ;
#26600=DIRECTION ( 'NONE',  ( -1.000000000000000000, 0.000000000000000000, 0.000000000000000000 ) ) ;
#26627=VECTOR ( 'NONE', #17337, 1000.000000000000000 ) ;
#26654=VECTOR ( 'NONE', #13521, 1000.000000000000000 ) ;
#26660=SHAPE_REPRESENTATION_RELATIONSHIP ( 'NONE' , 'NONE' ,  #24148, #29596 ) ;
#26691=CARTESIAN_POINT ( 'NONE',  ( 13.00000000000001243, 55.00000000000000711, 23.00000000000000000 ) ) ;
#26696=EDGE_LOOP ( 'NONE', ( #28214, #10591, #13233, #8807 ) ) ;
#26745=EDGE_CURVE ( 'NONE', #10204, #846, #18439, .T. ) ;
#26755=CARTESIAN_POINT ( 'NONE',  ( -5.000000000000000000, 0.000000000000000000, 23.00000000000000000 ) ) ;
#26773=ORIENTED_EDGE ( 'NONE', *, *, #9800, .F. ) ;
#26800=PLANE ( 'NONE',  #15026 ) ;
#26824=EDGE_CURVE ( 'NONE', #28903, #22806, #28227, .T. ) ;
#26870=CYLINDRICAL_SURFACE ( 'NONE', #1512, 5.000000000000000000 ) ;
#26896=ORIENTED_EDGE ( 'NONE', *, *, #17209, .F. ) ;
#26898=PRODUCT_DEFINITION ( 'UNKNOWN', '', #10719, #17704 ) ;
#26930=EDGE_LOOP ( 'NONE', ( #17836, #29336, #13561, #27909 ) ) ;
#26957=FACE_OUTER_BOUND ( 'NONE', #12196, .T. ) ;
#27084=PLANE ( 'NONE',  #3274 ) ;
#27112=ORIENTED_EDGE ( 'NONE', *, *, #15930, .T. ) ;
#27132=DIRECTION ( 'NONE',  ( 1.000000000000000000, 0.000000000000000000, 0.000000000000000000 ) ) ;
#27141=CYLINDRICAL_SURFACE ( 'NONE', #17326, 5.000000000000000888 ) ;
#27247=VERTEX_POINT ( 'NONE', #1812 ) ;
#27255=CARTESIAN_POINT ( 'NONE',  ( 13.00000000000000178, -2.870178842070716726E-15, -18.00000000000000000 ) ) ;
#27257=DIRECTION ( 'NONE',  ( -1.000000000000000000, 0.000000000000000000, 0.000000000000000000 ) ) ;
#27343=ORIENTED_EDGE ( 'NONE', *, *, #21561, .F. ) ;
#27371=AXIS2_PLACEMENT_3D ( 'NONE', #17016, #553, #28654 ) ;
#27376=EDGE_LOOP ( 'NONE', ( #3291, #20803, #11170, #12816 ) ) ;
#27383=DIRECTION ( 'NONE',  ( 1.000000000000000000, 0.000000000000000000, 0.000000000000000000 ) ) ;
#27390=VERTEX_POINT ( 'NONE', #25004 ) ;
#27399=ADVANCED_FACE ( 'NONE', ( #21738, #26957, #17160 ), #26800, .F. ) ;
#27463=ORIENTED_EDGE ( 'NONE', *, *, #9296, .F. ) ;
#27464=CARTESIAN_POINT ( 'NONE',  ( 0.000000000000000000, 0.000000000000000000, -23.00000000000000000 ) ) ;
#27478=EDGE_LOOP ( 'NONE', ( #19858, #11744, #7673, #18409 ) ) ;
#27497=LINE ( 'NONE', #6704, #27845 ) ;
#27557=DIRECTION ( 'NONE',  ( -0.000000000000000000, -1.000000000000000000, -0.000000000000000000 ) ) ;
#27572=VECTOR ( 'NONE', #5217, 1000.000000000000000 ) ;
#27576=CYLINDRICAL_SURFACE ( 'NONE', #820, 5.000000000000000888 ) ;
#27580=VERTEX_POINT ( 'NONE', #5570 ) ;
#27583=CARTESIAN_POINT ( 'NONE',  ( -0.000000000000000000, 55.00000000000000711, 18.00000000000000000 ) ) ;
#27594=DIRECTION ( 'NONE',  ( 0.000000000000000000, -1.000000000000000000, 0.000000000000000000 ) ) ;
#27648=DIRECTION ( 'NONE',  ( 0.000000000000000000, -1.000000000000000000, -0.000000000000000000 ) ) ;
#27665=AXIS2_PLACEMENT_3D ( 'NONE', #2527, #19268, #25861 ) ;
#27733=ORIENTED_EDGE ( 'NONE', *, *, #1837, .F. ) ;
#27808=AXIS2_PLACEMENT_3D ( 'NONE', #3613, #873, #3463 ) ;
#27845=VECTOR ( 'NONE', #4112, 1000.000000000000000 ) ;
#27857=DIRECTION ( 'NONE',  ( 1.000000000000000000, 0.000000000000000000, 0.000000000000000000 ) ) ;
#27889=AXIS2_PLACEMENT_3D ( 'NONE', #7563, #16865, #9987 ) ;
#27909=ORIENTED_EDGE ( 'NONE', *, *, #8951, .T. ) ;
#27929=VERTEX_POINT ( 'NONE', #3285 ) ;
#28002=CIRCLE ( 'NONE', #19197, 5.000000000000000000 ) ;
#28007=CARTESIAN_POINT ( 'NONE',  ( -13.00000000000000178, -2.870178842070716726E-15, 18.00000000000000000 ) ) ;
#28054=ORIENTED_EDGE ( 'NONE', *, *, #17914, .F. ) ;
#28141=ORIENTED_EDGE ( 'NONE', *, *, #18133, .F. ) ;
#28214=ORIENTED_EDGE ( 'NONE', *, *, #8323, .F. ) ;
#28227=CIRCLE ( 'NONE', #9164, 5.000000000000000888 ) ;
#28277=ORIENTED_EDGE ( 'NONE', *, *, #18728, .T. ) ;
#28367=CARTESIAN_POINT ( 'NONE',  ( 20.00000000000000355, 60.00000000000000711, -24.99999999999999645 ) ) ;
#28462=CARTESIAN_POINT ( 'NONE',  ( -13.00000000000001243, 55.00000000000000711, -18.00000000000000000 ) ) ;
#28463=ORIENTED_EDGE ( 'NONE', *, *, #26563, .T. ) ;
#28472=DIRECTION ( 'NONE',  ( -2.207829878515935943E-16, 1.000000000000000000, 0.000000000000000000 ) ) ;
#28489=ORIENTED_EDGE ( 'NONE', *, *, #20237, .T. ) ;
#28514=PLANE ( 'NONE',  #27889 ) ;
#28542=DIRECTION ( 'NONE',  ( 0.000000000000000000, 0.000000000000000000, 1.000000000000000000 ) ) ;
#28546=EDGE_CURVE ( 'NONE', #29924, #17091, #12155, .T. ) ;
#28566=AXIS2_PLACEMENT_3D ( 'NONE', #790, #2793, #19394 ) ;
#28575=DIRECTION ( 'NONE',  ( -0.000000000000000000, -0.000000000000000000, 1.000000000000000000 ) ) ;
#28614=FACE_OUTER_BOUND ( 'NONE', #6118, .T. ) ;
#28626=DIRECTION ( 'NONE',  ( 1.000000000000000000, 0.000000000000000000, 0.000000000000000000 ) ) ;
#28654=DIRECTION ( 'NONE',  ( 0.000000000000000000, 0.000000000000000000, -1.000000000000000000 ) ) ;
#28674=VERTEX_POINT ( 'NONE', #4432 ) ;
#28745=LINE ( 'NONE', #26424, #18417 ) ;
#28799=VECTOR ( 'NONE', #27132, 1000.000000000000000 ) ;
#28844=EDGE_CURVE ( 'NONE', #28674, #25189, #7773, .T. ) ;
#28903=VERTEX_POINT ( 'NONE', #752 ) ;
#28919=LINE ( 'NONE', #26755, #9466 ) ;
#28946=CARTESIAN_POINT ( 'NONE',  ( 8.500000000000088818, 17.32050807568872486, -23.00000000000000000 ) ) ;
#29091=CARTESIAN_POINT ( 'NONE',  ( -5.000000000000000000, 0.000000000000000000, -23.00000000000000000 ) ) ;
#29096=DIRECTION ( 'NONE',  ( -1.000000000000000000, 2.207829878515935943E-16, 0.000000000000000000 ) ) ;
#29139=CIRCLE ( 'NONE', #16849, 1.499999999999996225 ) ;
#29198=ORIENTED_EDGE ( 'NONE', *, *, #18578, .F. ) ;
#29336=ORIENTED_EDGE ( 'NONE', *, *, #24742, .F. ) ;
#29415=AXIS2_PLACEMENT_3D ( 'NONE', #20769, #22784, #2341 ) ;
#29425=CIRCLE ( 'NONE', #21084, 5.000000000000000000 ) ;
#29450=ORIENTED_EDGE ( 'NONE', *, *, #15722, .F. ) ;
#29476=VECTOR ( 'NONE', #23268, 1000.000000000000000 ) ;
#29490=DIRECTION ( 'NONE',  ( -0.000000000000000000, 1.000000000000000000, -0.000000000000000000 ) ) ;
#29513=CARTESIAN_POINT ( 'NONE',  ( 20.00000000000000355, 55.00000000000000711, -24.99999999999999645 ) ) ;
#29533=EDGE_CURVE ( 'NONE', #22806, #29940, #6810, .T. ) ;
#29543=VERTEX_POINT ( 'NONE', #16104 ) ;
#29592=VERTEX_POINT ( 'NONE', #13221 ) ;
#29596=ADVANCED_BREP_SHAPE_REPRESENTATION ( '', ( #21231, #13190 ), #3942 ) ;
#29597=ORIENTED_EDGE ( 'NONE', *, *, #26323, .T. ) ;
#29679=DIRECTION ( 'NONE',  ( 1.000000000000000000, 0.000000000000000000, 0.000000000000000000 ) ) ;
#29704=DIRECTION ( 'NONE',  ( 0.000000000000000000, -1.000000000000000000, 0.000000000000000000 ) ) ;
#29816=ORIENTED_EDGE ( 'NONE', *, *, #951, .T. ) ;
#29821=VECTOR ( 'NONE', #1791, 1000.000000000000000 ) ;
#29859=CARTESIAN_POINT ( 'NONE',  ( -5.000000000000000000, 0.000000000000000000, 23.00000000000000000 ) ) ;
#29867=ORIENTED_EDGE ( 'NONE', *, *, #20621, .F. ) ;
#29870=DIRECTION ( 'NONE',  ( 2.207829878515935943E-16, 1.000000000000000000, 0.000000000000000000 ) ) ;
#29904=LINE ( 'NONE', #18534, #19654 ) ;
#29924=VERTEX_POINT ( 'NONE', #16620 ) ;
#29940=VERTEX_POINT ( 'NONE', #19058 ) ;
#29957=ORIENTED_EDGE ( 'NONE', *, *, #15522, .F. ) ;
#29979=EDGE_LOOP ( 'NONE', ( #4162, #9499, #20902, #20575 ) ) ;
#29980=EDGE_LOOP ( 'NONE', ( #21073, #852, #19576, #25825, #5647, #15466, #24667, #13767 ) ) ;
#29986=ORIENTED_EDGE ( 'NONE', *, *, #11689, .T. ) ;
#30003=CARTESIAN_POINT ( 'NONE',  ( -19.99999999999998934, 60.00000000000000711, 29.99999999999999289 ) ) ;
#30006=EDGE_LOOP ( 'NONE', ( #9748, #27112, #8125, #24218 ) ) ;
#30007=PLANE ( 'NONE',  #29415 ) ;
#30012=UNCERTAINTY_MEASURE_WITH_UNIT (LENGTH_MEASURE( 1.000000000000000082E-05 ), #3163, 'distance_accuracy_value', 'NONE');
#30063=ADVANCED_FACE ( 'NONE', ( #1362 ), #26870, .F. ) ;
#30090=DIRECTION ( 'NONE',  ( -0.000000000000000000, -0.000000000000000000, 1.000000000000000000 ) ) ;
#30102=CARTESIAN_POINT ( 'NONE',  ( -13.00000000000000178, -2.870178842070716726E-15, -23.00000000000000000 ) ) ;
#30129=VERTEX_POINT ( 'NONE', #8053 ) ;
#30130=ORIENTED_EDGE ( 'NONE', *, *, #3862, .T. ) ;
#30152=LINE ( 'NONE', #6906, #18621 ) ;
ENDSEC;
END-ISO-10303-21;
